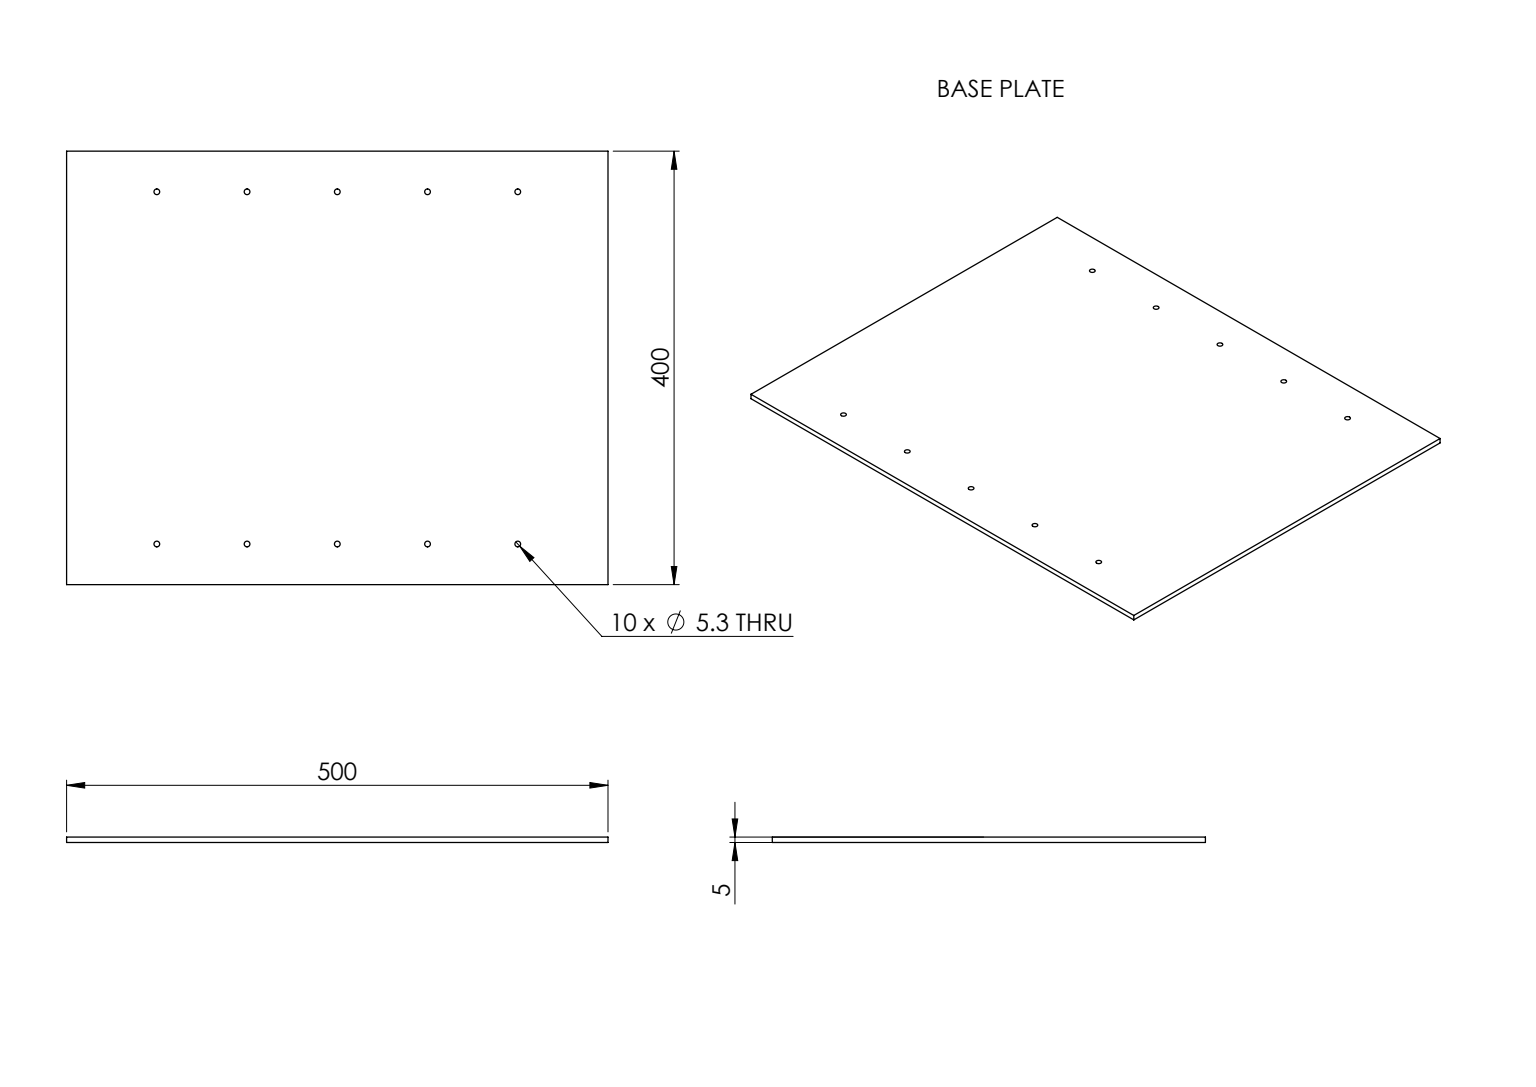
ISO-10303-21;
HEADER;
FILE_DESCRIPTION (('STEP AP214'),
    '1' );
FILE_NAME ('base plate.step',
    '2026-10-24T14:05:44',
    ( '' ),
    ( '' ),
    'SwSTEP 2.0',
    'SolidWorks 2026',
    '' );
FILE_SCHEMA (( 'AUTOMOTIVE_DESIGN' ));
ENDSEC;

DATA;
#1=ORIENTED_EDGE ( 'NONE', *, *, #3686, .F. ) ;
#8=CARTESIAN_POINT ( 'NONE',  ( 53.33333333333330017, -20.00000000000000000, -165.1500000000000625 ) ) ;
#40=ORIENTED_EDGE ( 'NONE', *, *, #976, .T. ) ;
#60=EDGE_LOOP ( 'NONE', ( #5047, #1369, #5230, #2362 ) ) ;
#62=FACE_OUTER_BOUND ( 'NONE', #5362, .T. ) ;
#64=AXIS2_PLACEMENT_3D ( 'NONE', #2945, #3017, #209 ) ;
#88=DIRECTION ( 'NONE',  ( -0.000000000000000000, 1.000000000000000000, -0.000000000000000000 ) ) ;
#107=EDGE_LOOP ( 'NONE', ( #5090, #2760, #2727, #2223 ) ) ;
#119=DIRECTION ( 'NONE',  ( 0.000000000000000000, 0.000000000000000000, 1.000000000000000000 ) ) ;
#126=EDGE_LOOP ( 'NONE', ( #4642, #4899, #6680, #3898 ) ) ;
#139=DIRECTION ( 'NONE',  ( -0.000000000000000000, -1.000000000000000000, -0.000000000000000000 ) ) ;
#143=ADVANCED_FACE ( 'NONE', ( #298 ), #1009, .F. ) ;
#147=EDGE_LOOP ( 'NONE', ( #2986, #2941 ) ) ;
#150=EDGE_CURVE ( 'NONE', #1987, #1784, #6703, .T. ) ;
#153=VERTEX_POINT ( 'NONE', #2555 ) ;
#179=ORIENTED_EDGE ( 'NONE', *, *, #5269, .F. ) ;
#209=DIRECTION ( 'NONE',  ( 0.000000000000000000, 0.000000000000000000, 1.000000000000000000 ) ) ;
#219=ORIENTED_EDGE ( 'NONE', *, *, #5940, .T. ) ;
#235=EDGE_CURVE ( 'NONE', #4841, #4123, #4707, .T. ) ;
#243=DIRECTION ( 'NONE',  ( -0.000000000000000000, -1.000000000000000000, -0.000000000000000000 ) ) ;
#260=EDGE_CURVE ( 'NONE', #6697, #3198, #4705, .T. ) ;
#267=CARTESIAN_POINT ( 'NONE',  ( -30.00000000000002842, -25.00000000000000000, 200.0000000000000000 ) ) ;
#271=VERTEX_POINT ( 'NONE', #4467 ) ;
#277=VECTOR ( 'NONE', #2807, 1000.000000000000000 ) ;
#283=CARTESIAN_POINT ( 'NONE',  ( 219.9999999999999716, -25.00000000000000000, -165.1500000000000625 ) ) ;
#285=CARTESIAN_POINT ( 'NONE',  ( 303.3333333333333144, -25.00000000000000000, -162.5000000000000853 ) ) ;
#287=( NAMED_UNIT ( * ) SI_UNIT ( $, .STERADIAN. ) SOLID_ANGLE_UNIT ( ) );
#298=FACE_OUTER_BOUND ( 'NONE', #2619, .T. ) ;
#302=LINE ( 'NONE', #894, #3741 ) ;
#303=CYLINDRICAL_SURFACE ( 'NONE', #4799, 2.649999999999985700 ) ;
#312=ORIENTED_EDGE ( 'NONE', *, *, #4187, .T. ) ;
#317=CARTESIAN_POINT ( 'NONE',  ( 386.6666666666666288, -20.00000000000000000, 165.1500000000000625 ) ) ;
#333=EDGE_LOOP ( 'NONE', ( #4442, #2385, #6375, #2319 ) ) ;
#334=( GEOMETRIC_REPRESENTATION_CONTEXT ( 3 ) GLOBAL_UNCERTAINTY_ASSIGNED_CONTEXT ( ( #6417 ) ) GLOBAL_UNIT_ASSIGNED_CONTEXT ( ( #4283, #1950, #1436 ) ) REPRESENTATION_CONTEXT ( 'NONE', 'WORKASPACE' ) );
#337=EDGE_CURVE ( 'NONE', #6618, #3696, #5673, .T. ) ;
#338=ORIENTED_EDGE ( 'NONE', *, *, #2679, .T. ) ;
#344=CARTESIAN_POINT ( 'NONE',  ( 136.6666666666666288, -20.00000000000000000, 165.1500000000000625 ) ) ;
#346=CYLINDRICAL_SURFACE ( 'NONE', #6243, 2.649999999999985700 ) ;
#348=EDGE_LOOP ( 'NONE', ( #1624, #5425 ) ) ;
#354=DIRECTION ( 'NONE',  ( 0.000000000000000000, 0.000000000000000000, -1.000000000000000000 ) ) ;
#366=ORIENTED_EDGE ( 'NONE', *, *, #235, .T. ) ;
#381=FACE_OUTER_BOUND ( 'NONE', #2480, .T. ) ;
#391=CARTESIAN_POINT ( 'NONE',  ( -30.00000000000002842, -25.00000000000000000, 200.0000000000000000 ) ) ;
#403=DIRECTION ( 'NONE',  ( -0.000000000000000000, -1.000000000000000000, -0.000000000000000000 ) ) ;
#416=EDGE_CURVE ( 'NONE', #2352, #4993, #2170, .T. ) ;
#420=AXIS2_PLACEMENT_3D ( 'NONE', #1513, #3788, #1169 ) ;
#421=AXIS2_PLACEMENT_3D ( 'NONE', #5145, #5665, #2248 ) ;
#430=EDGE_CURVE ( 'NONE', #5253, #5386, #3873, .T. ) ;
#432=VERTEX_POINT ( 'NONE', #3020 ) ;
#438=CARTESIAN_POINT ( 'NONE',  ( 219.9999999999999716, -20.00000000000000000, -165.1500000000000625 ) ) ;
#440=EDGE_CURVE ( 'NONE', #3349, #7332, #2788, .T. ) ;
#450=VERTEX_POINT ( 'NONE', #1982 ) ;
#459=AXIS2_PLACEMENT_3D ( 'NONE', #4842, #4603, #3459 ) ;
#460=CARTESIAN_POINT ( 'NONE',  ( -30.00000000000002842, -20.00000000000000000, 200.0000000000000000 ) ) ;
#462=EDGE_CURVE ( 'NONE', #1179, #5999, #4944, .T. ) ;
#473=DIRECTION ( 'NONE',  ( 0.000000000000000000, 1.000000000000000000, 0.000000000000000000 ) ) ;
#488=EDGE_LOOP ( 'NONE', ( #3716, #3762 ) ) ;
#513=LINE ( 'NONE', #4964, #4728 ) ;
#517=AXIS2_PLACEMENT_3D ( 'NONE', #2143, #842, #1959 ) ;
#521=EDGE_CURVE ( 'NONE', #1652, #1784, #3123, .T. ) ;
#526=DIRECTION ( 'NONE',  ( -0.000000000000000000, -1.000000000000000000, -0.000000000000000000 ) ) ;
#541=VERTEX_POINT ( 'NONE', #1871 ) ;
#546=AXIS2_PLACEMENT_3D ( 'NONE', #3740, #473, #7159 ) ;
#570=ORIENTED_EDGE ( 'NONE', *, *, #1823, .T. ) ;
#578=ORIENTED_EDGE ( 'NONE', *, *, #7274, .F. ) ;
#579=DIRECTION ( 'NONE',  ( -0.000000000000000000, 1.000000000000000000, -0.000000000000000000 ) ) ;
#582=CARTESIAN_POINT ( 'NONE',  ( 136.6666666666666288, -20.00000000000000000, 162.5000000000000853 ) ) ;
#585=DIRECTION ( 'NONE',  ( 0.000000000000000000, 0.000000000000000000, -1.000000000000000000 ) ) ;
#587=DIRECTION ( 'NONE',  ( -0.000000000000000000, 1.000000000000000000, -0.000000000000000000 ) ) ;
#600=DIRECTION ( 'NONE',  ( -0.000000000000000000, -1.000000000000000000, -0.000000000000000000 ) ) ;
#625=SHAPE_DEFINITION_REPRESENTATION ( #940, #4771 ) ;
#628=DIRECTION ( 'NONE',  ( 0.000000000000000000, 0.000000000000000000, 1.000000000000000000 ) ) ;
#641=ORIENTED_EDGE ( 'NONE', *, *, #1393, .T. ) ;
#647=VERTEX_POINT ( 'NONE', #6436 ) ;
#653=ORIENTED_EDGE ( 'NONE', *, *, #416, .T. ) ;
#658=DIRECTION ( 'NONE',  ( 0.000000000000000000, 0.000000000000000000, -1.000000000000000000 ) ) ;
#659=DIRECTION ( 'NONE',  ( 0.000000000000000000, 1.000000000000000000, 0.000000000000000000 ) ) ;
#672=AXIS2_PLACEMENT_3D ( 'NONE', #2662, #4518, #2775 ) ;
#674=CARTESIAN_POINT ( 'NONE',  ( -30.00000000000002842, -20.00000000000000000, 200.0000000000000000 ) ) ;
#680=EDGE_CURVE ( 'NONE', #5556, #1411, #5423, .T. ) ;
#695=DIRECTION ( 'NONE',  ( 0.000000000000000000, 0.000000000000000000, 1.000000000000000000 ) ) ;
#706=DIRECTION ( 'NONE',  ( 0.000000000000000000, 1.000000000000000000, 0.000000000000000000 ) ) ;
#723=DIRECTION ( 'NONE',  ( -0.000000000000000000, 1.000000000000000000, -0.000000000000000000 ) ) ;
#758=AXIS2_PLACEMENT_3D ( 'NONE', #4531, #139, #4493 ) ;
#763=VERTEX_POINT ( 'NONE', #2931 ) ;
#786=DIRECTION ( 'NONE',  ( -0.000000000000000000, -1.000000000000000000, -0.000000000000000000 ) ) ;
#791=ORIENTED_EDGE ( 'NONE', *, *, #2057, .T. ) ;
#793=CARTESIAN_POINT ( 'NONE',  ( -30.00000000000002842, -20.00000000000000000, 200.0000000000000000 ) ) ;
#795=ORIENTED_EDGE ( 'NONE', *, *, #7297, .F. ) ;
#796=AXIS2_PLACEMENT_3D ( 'NONE', #1331, #817, #2406 ) ;
#799=CARTESIAN_POINT ( 'NONE',  ( 136.6666666666666288, -20.00000000000000000, -162.5000000000000853 ) ) ;
#802=CARTESIAN_POINT ( 'NONE',  ( 53.33333333333330017, -25.00000000000000000, -159.8500000000001080 ) ) ;
#803=DIRECTION ( 'NONE',  ( 0.000000000000000000, 1.000000000000000000, 0.000000000000000000 ) ) ;
#808=CARTESIAN_POINT ( 'NONE',  ( 53.33333333333330017, -20.00000000000000000, -162.5000000000000853 ) ) ;
#817=DIRECTION ( 'NONE',  ( -0.000000000000000000, -1.000000000000000000, -0.000000000000000000 ) ) ;
#822=DIRECTION ( 'NONE',  ( -0.000000000000000000, 1.000000000000000000, -0.000000000000000000 ) ) ;
#835=ORIENTED_EDGE ( 'NONE', *, *, #5690, .T. ) ;
#837=EDGE_LOOP ( 'NONE', ( #3025, #4554, #2784, #5893 ) ) ;
#842=DIRECTION ( 'NONE',  ( 0.000000000000000000, 1.000000000000000000, 0.000000000000000000 ) ) ;
#847=VERTEX_POINT ( 'NONE', #1917 ) ;
#849=EDGE_CURVE ( 'NONE', #1411, #5556, #4851, .T. ) ;
#858=ORIENTED_EDGE ( 'NONE', *, *, #5162, .T. ) ;
#867=DIRECTION ( 'NONE',  ( 0.000000000000000000, 1.000000000000000000, 0.000000000000000000 ) ) ;
#877=SURFACE_STYLE_USAGE ( .BOTH. , #6014 ) ;
#882=CARTESIAN_POINT ( 'NONE',  ( 386.6666666666666288, -25.00000000000000000, -159.8500000000001080 ) ) ;
#891=CIRCLE ( 'NONE', #4830, 2.649999999999985700 ) ;
#894=CARTESIAN_POINT ( 'NONE',  ( 470.0000000000000000, -20.00000000000000000, 200.0000000000000000 ) ) ;
#911=DIRECTION ( 'NONE',  ( -0.000000000000000000, 1.000000000000000000, -0.000000000000000000 ) ) ;
#912=DIRECTION ( 'NONE',  ( 0.000000000000000000, 0.000000000000000000, -1.000000000000000000 ) ) ;
#940=PRODUCT_DEFINITION_SHAPE ( 'NONE', 'NONE',  #1667 ) ;
#950=DIRECTION ( 'NONE',  ( 0.000000000000000000, 0.000000000000000000, -1.000000000000000000 ) ) ;
#976=EDGE_CURVE ( 'NONE', #1043, #7189, #7265, .T. ) ;
#979=AXIS2_PLACEMENT_3D ( 'NONE', #799, #3053, #4229 ) ;
#989=PRODUCT_DEFINITION_CONTEXT ( 'detailed design', #5793, 'design' ) ;
#996=CARTESIAN_POINT ( 'NONE',  ( 219.9999999999999716, -20.00000000000000000, 162.5000000000000853 ) ) ;
#1009=CYLINDRICAL_SURFACE ( 'NONE', #5553, 2.649999999999985700 ) ;
#1010=CARTESIAN_POINT ( 'NONE',  ( 136.6666666666666288, -25.00000000000000000, 162.5000000000000853 ) ) ;
#1015=FACE_BOUND ( 'NONE', #4450, .T. ) ;
#1018=EDGE_CURVE ( 'NONE', #1043, #3333, #7260, .T. ) ;
#1026=EDGE_CURVE ( 'NONE', #271, #6816, #6904, .T. ) ;
#1043=VERTEX_POINT ( 'NONE', #2156 ) ;
#1047=ORIENTED_EDGE ( 'NONE', *, *, #5906, .F. ) ;
#1050=DIRECTION ( 'NONE',  ( 0.000000000000000000, 0.000000000000000000, 1.000000000000000000 ) ) ;
#1054=DIRECTION ( 'NONE',  ( 0.000000000000000000, -0.000000000000000000, 1.000000000000000000 ) ) ;
#1062=ORIENTED_EDGE ( 'NONE', *, *, #6098, .T. ) ;
#1088=AXIS2_PLACEMENT_3D ( 'NONE', #3698, #5427, #3116 ) ;
#1097=LINE ( 'NONE', #3327, #6852 ) ;
#1116=DIRECTION ( 'NONE',  ( 0.000000000000000000, 1.000000000000000000, 0.000000000000000000 ) ) ;
#1119=ORIENTED_EDGE ( 'NONE', *, *, #5813, .F. ) ;
#1121=FACE_BOUND ( 'NONE', #5959, .T. ) ;
#1124=LINE ( 'NONE', #2758, #4238 ) ;
#1131=AXIS2_PLACEMENT_3D ( 'NONE', #6762, #7281, #1465 ) ;
#1134=DIRECTION ( 'NONE',  ( 0.000000000000000000, 1.000000000000000000, 0.000000000000000000 ) ) ;
#1137=CIRCLE ( 'NONE', #6395, 2.649999999999985700 ) ;
#1147=CYLINDRICAL_SURFACE ( 'NONE', #2971, 2.649999999999985700 ) ;
#1148=LINE ( 'NONE', #3417, #4961 ) ;
#1160=AXIS2_PLACEMENT_3D ( 'NONE', #2718, #526, #4490 ) ;
#1163=DIRECTION ( 'NONE',  ( 0.000000000000000000, 1.000000000000000000, 0.000000000000000000 ) ) ;
#1164=EDGE_CURVE ( 'NONE', #5386, #5253, #2926, .T. ) ;
#1169=DIRECTION ( 'NONE',  ( 0.000000000000000000, 0.000000000000000000, -1.000000000000000000 ) ) ;
#1174=DIRECTION ( 'NONE',  ( -0.000000000000000000, 1.000000000000000000, -0.000000000000000000 ) ) ;
#1177=ORIENTED_EDGE ( 'NONE', *, *, #6890, .F. ) ;
#1179=VERTEX_POINT ( 'NONE', #4139 ) ;
#1188=ORIENTED_EDGE ( 'NONE', *, *, #5813, .T. ) ;
#1206=ADVANCED_FACE ( 'NONE', ( #4742 ), #2925, .F. ) ;
#1236=ORIENTED_EDGE ( 'NONE', *, *, #5982, .F. ) ;
#1247=FACE_OUTER_BOUND ( 'NONE', #4443, .T. ) ;
#1258=VECTOR ( 'NONE', #3930, 1000.000000000000000 ) ;
#1261=ORIENTED_EDGE ( 'NONE', *, *, #6825, .F. ) ;
#1269=LINE ( 'NONE', #5767, #1561 ) ;
#1271=LINE ( 'NONE', #3538, #7254 ) ;
#1275=ADVANCED_FACE ( 'NONE', ( #4172 ), #5757, .T. ) ;
#1331=CARTESIAN_POINT ( 'NONE',  ( 386.6666666666666288, -25.00000000000000000, -162.5000000000000853 ) ) ;
#1338=DIRECTION ( 'NONE',  ( 0.000000000000000000, 1.000000000000000000, 0.000000000000000000 ) ) ;
#1340=ORIENTED_EDGE ( 'NONE', *, *, #1164, .T. ) ;
#1347=CARTESIAN_POINT ( 'NONE',  ( 219.9999999999999716, -20.00000000000000000, 165.1500000000000625 ) ) ;
#1349=DIRECTION ( 'NONE',  ( 0.000000000000000000, 0.000000000000000000, 1.000000000000000000 ) ) ;
#1366=UNCERTAINTY_MEASURE_WITH_UNIT (LENGTH_MEASURE( 1.000000000000000082E-05 ), #2021, 'distance_accuracy_value', 'NONE');
#1369=ORIENTED_EDGE ( 'NONE', *, *, #2451, .T. ) ;
#1379=FACE_OUTER_BOUND ( 'NONE', #3006, .T. ) ;
#1393=EDGE_CURVE ( 'NONE', #4485, #3484, #3897, .T. ) ;
#1411=VERTEX_POINT ( 'NONE', #882 ) ;
#1423=EDGE_CURVE ( 'NONE', #3349, #4841, #1557, .T. ) ;
#1424=FACE_OUTER_BOUND ( 'NONE', #3457, .T. ) ;
#1436=( NAMED_UNIT ( * ) SI_UNIT ( $, .STERADIAN. ) SOLID_ANGLE_UNIT ( ) );
#1438=DIRECTION ( 'NONE',  ( 0.000000000000000000, 0.000000000000000000, -1.000000000000000000 ) ) ;
#1446=EDGE_LOOP ( 'NONE', ( #4100, #4125, #4120, #7273 ) ) ;
#1449=CARTESIAN_POINT ( 'NONE',  ( 219.9999999999999716, -20.00000000000000000, 162.5000000000000853 ) ) ;
#1453=EDGE_CURVE ( 'NONE', #2910, #7189, #2090, .T. ) ;
#1456=ORIENTED_EDGE ( 'NONE', *, *, #5758, .T. ) ;
#1465=DIRECTION ( 'NONE',  ( 0.000000000000000000, 0.000000000000000000, -1.000000000000000000 ) ) ;
#1466=EDGE_CURVE ( 'NONE', #647, #3098, #2439, .T. ) ;
#1478=AXIS2_PLACEMENT_3D ( 'NONE', #460, #1163, #1054 ) ;
#1499=VECTOR ( 'NONE', #3835, 1000.000000000000000 ) ;
#1501=FACE_BOUND ( 'NONE', #6434, .T. ) ;
#1504=ORIENTED_EDGE ( 'NONE', *, *, #4187, .F. ) ;
#1508=CARTESIAN_POINT ( 'NONE',  ( 303.3333333333333144, -20.00000000000000000, -159.8500000000001080 ) ) ;
#1510=EDGE_CURVE ( 'NONE', #4492, #3944, #513, .T. ) ;
#1513=CARTESIAN_POINT ( 'NONE',  ( 386.6666666666666288, -25.00000000000000000, -162.5000000000000853 ) ) ;
#1515=EDGE_LOOP ( 'NONE', ( #2970, #4408 ) ) ;
#1533=ORIENTED_EDGE ( 'NONE', *, *, #2575, .F. ) ;
#1540=ORIENTED_EDGE ( 'NONE', *, *, #235, .F. ) ;
#1557=LINE ( 'NONE', #4406, #1499 ) ;
#1561=VECTOR ( 'NONE', #7037, 1000.000000000000000 ) ;
#1569=AXIS2_PLACEMENT_3D ( 'NONE', #7251, #7325, #5370 ) ;
#1577=ORIENTED_EDGE ( 'NONE', *, *, #3686, .T. ) ;
#1578=ORIENTED_EDGE ( 'NONE', *, *, #3283, .T. ) ;
#1585=DIRECTION ( 'NONE',  ( -0.000000000000000000, -1.000000000000000000, -0.000000000000000000 ) ) ;
#1587=VECTOR ( 'NONE', #3164, 1000.000000000000000 ) ;
#1599=CARTESIAN_POINT ( 'NONE',  ( -30.00000000000002842, -25.00000000000000000, -200.0000000000000000 ) ) ;
#1600=ADVANCED_FACE ( 'NONE', ( #5040 ), #5631, .F. ) ;
#1603=AXIS2_PLACEMENT_3D ( 'NONE', #2576, #2138, #7243 ) ;
#1614=ORIENTED_EDGE ( 'NONE', *, *, #2679, .F. ) ;
#1624=ORIENTED_EDGE ( 'NONE', *, *, #337, .T. ) ;
#1643=CIRCLE ( 'NONE', #2578, 2.649999999999985700 ) ;
#1644=DIRECTION ( 'NONE',  ( 0.000000000000000000, 0.000000000000000000, 1.000000000000000000 ) ) ;
#1652=VERTEX_POINT ( 'NONE', #6346 ) ;
#1663=CARTESIAN_POINT ( 'NONE',  ( 53.33333333333330017, -20.00000000000000000, 162.5000000000000853 ) ) ;
#1667=PRODUCT_DEFINITION ( 'UNKNOWN', '', #5185, #989 ) ;
#1687=LINE ( 'NONE', #6264, #5936 ) ;
#1695=DIRECTION ( 'NONE',  ( -0.000000000000000000, 1.000000000000000000, -0.000000000000000000 ) ) ;
#1697=CARTESIAN_POINT ( 'NONE',  ( 219.9999999999999716, -20.00000000000000000, -162.5000000000000853 ) ) ;
#1709=ORIENTED_EDGE ( 'NONE', *, *, #1466, .T. ) ;
#1711=DIRECTION ( 'NONE',  ( 0.000000000000000000, 1.000000000000000000, 0.000000000000000000 ) ) ;
#1729=DIRECTION ( 'NONE',  ( 0.000000000000000000, 1.000000000000000000, 0.000000000000000000 ) ) ;
#1730=EDGE_CURVE ( 'NONE', #5656, #6176, #4084, .T. ) ;
#1740=CARTESIAN_POINT ( 'NONE',  ( -30.00000000000002842, -25.00000000000000000, -200.0000000000000000 ) ) ;
#1746=VECTOR ( 'NONE', #2696, 1000.000000000000000 ) ;
#1748=DIRECTION ( 'NONE',  ( 0.000000000000000000, 0.000000000000000000, 1.000000000000000000 ) ) ;
#1761=ORIENTED_EDGE ( 'NONE', *, *, #6890, .T. ) ;
#1764=DIRECTION ( 'NONE',  ( 0.000000000000000000, 0.000000000000000000, 1.000000000000000000 ) ) ;
#1767=CARTESIAN_POINT ( 'NONE',  ( 136.6666666666666288, -20.00000000000000000, 165.1500000000000625 ) ) ;
#1772=VERTEX_POINT ( 'NONE', #6001 ) ;
#1784=VERTEX_POINT ( 'NONE', #1347 ) ;
#1796=VECTOR ( 'NONE', #7286, 1000.000000000000000 ) ;
#1800=EDGE_CURVE ( 'NONE', #6816, #271, #7127, .T. ) ;
#1803=ORIENTED_EDGE ( 'NONE', *, *, #462, .T. ) ;
#1814=ORIENTED_EDGE ( 'NONE', *, *, #1800, .F. ) ;
#1823=EDGE_CURVE ( 'NONE', #3661, #5128, #4733, .T. ) ;
#1845=AXIS2_PLACEMENT_3D ( 'NONE', #4035, #706, #5800 ) ;
#1860=DIRECTION ( 'NONE',  ( -0.000000000000000000, -1.000000000000000000, -0.000000000000000000 ) ) ;
#1864=EDGE_CURVE ( 'NONE', #7332, #4123, #7277, .T. ) ;
#1871=CARTESIAN_POINT ( 'NONE',  ( 386.6666666666666288, -25.00000000000000000, 159.8500000000001080 ) ) ;
#1895=CARTESIAN_POINT ( 'NONE',  ( 303.3333333333333144, -20.00000000000000000, 159.8500000000001080 ) ) ;
#1898=DIRECTION ( 'NONE',  ( -0.000000000000000000, -1.000000000000000000, -0.000000000000000000 ) ) ;
#1900=CIRCLE ( 'NONE', #6115, 2.649999999999985700 ) ;
#1912=ORIENTED_EDGE ( 'NONE', *, *, #1423, .F. ) ;
#1914=CARTESIAN_POINT ( 'NONE',  ( -30.00000000000002842, -25.00000000000000000, 200.0000000000000000 ) ) ;
#1915=AXIS2_PLACEMENT_3D ( 'NONE', #2600, #4262, #4858 ) ;
#1917=CARTESIAN_POINT ( 'NONE',  ( 53.33333333333330017, -20.00000000000000000, 165.1500000000000625 ) ) ;
#1943=APPLICATION_CONTEXT ( 'automotive_design' ) ;
#1950=( NAMED_UNIT ( * ) PLANE_ANGLE_UNIT ( ) SI_UNIT ( $, .RADIAN. ) );
#1951=FILL_AREA_STYLE ('',( #2546 ) ) ;
#1953=MECHANICAL_DESIGN_GEOMETRIC_PRESENTATION_REPRESENTATION('',(#3392),#4358);
#1959=DIRECTION ( 'NONE',  ( 0.000000000000000000, 0.000000000000000000, -1.000000000000000000 ) ) ;
#1961=ORIENTED_EDGE ( 'NONE', *, *, #5344, .T. ) ;
#1963=AXIS2_PLACEMENT_3D ( 'NONE', #2294, #628, #5829 ) ;
#1970=CYLINDRICAL_SURFACE ( 'NONE', #2320, 2.649999999999985700 ) ;
#1977=PLANE ( 'NONE',  #1088 ) ;
#1980=DIRECTION ( 'NONE',  ( 0.000000000000000000, 1.000000000000000000, 0.000000000000000000 ) ) ;
#1982=CARTESIAN_POINT ( 'NONE',  ( 386.6666666666666288, -25.00000000000000000, 165.1500000000000625 ) ) ;
#1987=VERTEX_POINT ( 'NONE', #4676 ) ;
#1999=ORIENTED_EDGE ( 'NONE', *, *, #6583, .F. ) ;
#2010=CARTESIAN_POINT ( 'NONE',  ( 303.3333333333333144, -20.00000000000000000, -162.5000000000000853 ) ) ;
#2012=FACE_OUTER_BOUND ( 'NONE', #6212, .T. ) ;
#2021=( LENGTH_UNIT ( ) NAMED_UNIT ( * ) SI_UNIT ( .MILLI., .METRE. ) );
#2029=PLANE ( 'NONE',  #6297 ) ;
#2037=DIRECTION ( 'NONE',  ( 0.000000000000000000, 0.000000000000000000, -1.000000000000000000 ) ) ;
#2040=CARTESIAN_POINT ( 'NONE',  ( 53.33333333333330017, -20.00000000000000000, 162.5000000000000853 ) ) ;
#2046=EDGE_CURVE ( 'NONE', #647, #7294, #1271, .T. ) ;
#2057=EDGE_CURVE ( 'NONE', #5128, #6618, #1687, .T. ) ;
#2060=CARTESIAN_POINT ( 'NONE',  ( -30.00000000000002842, -20.00000000000000000, 200.0000000000000000 ) ) ;
#2075=CIRCLE ( 'NONE', #6508, 2.649999999999985700 ) ;
#2090=CIRCLE ( 'NONE', #672, 2.649999999999985700 ) ;
#2092=FACE_BOUND ( 'NONE', #2505, .T. ) ;
#2104=EDGE_CURVE ( 'NONE', #2352, #2399, #3287, .T. ) ;
#2113=DIRECTION ( 'NONE',  ( -0.000000000000000000, 1.000000000000000000, -0.000000000000000000 ) ) ;
#2123=LINE ( 'NONE', #8, #6736 ) ;
#2132=EDGE_LOOP ( 'NONE', ( #578, #5329, #6288, #6562 ) ) ;
#2135=CARTESIAN_POINT ( 'NONE',  ( 219.9999999999999716, -25.00000000000000000, 162.5000000000000853 ) ) ;
#2137=DIRECTION ( 'NONE',  ( -0.000000000000000000, -0.000000000000000000, -1.000000000000000000 ) ) ;
#2138=DIRECTION ( 'NONE',  ( -0.000000000000000000, 1.000000000000000000, -0.000000000000000000 ) ) ;
#2139=ORIENTED_EDGE ( 'NONE', *, *, #5690, .F. ) ;
#2143=CARTESIAN_POINT ( 'NONE',  ( 219.9999999999999716, -20.00000000000000000, -162.5000000000000853 ) ) ;
#2145=( LENGTH_UNIT ( ) NAMED_UNIT ( * ) SI_UNIT ( .MILLI., .METRE. ) );
#2146=CYLINDRICAL_SURFACE ( 'NONE', #5290, 2.649999999999985700 ) ;
#2147=ORIENTED_EDGE ( 'NONE', *, *, #5344, .F. ) ;
#2149=EDGE_CURVE ( 'NONE', #3484, #4485, #5187, .T. ) ;
#2153=CARTESIAN_POINT ( 'NONE',  ( 303.3333333333333144, -25.00000000000000000, 165.1500000000000625 ) ) ;
#2156=CARTESIAN_POINT ( 'NONE',  ( 136.6666666666666288, -25.00000000000000000, 159.8500000000001080 ) ) ;
#2159=PLANE ( 'NONE',  #1478 ) ;
#2170=LINE ( 'NONE', #438, #6628 ) ;
#2189=AXIS2_PLACEMENT_3D ( 'NONE', #6987, #4093, #2950 ) ;
#2195=CARTESIAN_POINT ( 'NONE',  ( 386.6666666666666288, -20.00000000000000000, 162.5000000000000853 ) ) ;
#2196=CARTESIAN_POINT ( 'NONE',  ( 386.6666666666666288, -25.00000000000000000, -165.1500000000000625 ) ) ;
#2201=AXIS2_PLACEMENT_3D ( 'NONE', #2040, #822, #6674 ) ;
#2215=ORIENTED_EDGE ( 'NONE', *, *, #2149, .F. ) ;
#2216=AXIS2_PLACEMENT_3D ( 'NONE', #6208, #6238, #5117 ) ;
#2223=ORIENTED_EDGE ( 'NONE', *, *, #5444, .T. ) ;
#2224=ORIENTED_EDGE ( 'NONE', *, *, #4880, .F. ) ;
#2242=ADVANCED_FACE ( 'NONE', ( #3596 ), #4135, .F. ) ;
#2248=DIRECTION ( 'NONE',  ( 0.000000000000000000, 0.000000000000000000, 1.000000000000000000 ) ) ;
#2251=CARTESIAN_POINT ( 'NONE',  ( 386.6666666666666288, -20.00000000000000000, -162.5000000000000853 ) ) ;
#2268=EDGE_CURVE ( 'NONE', #7332, #3349, #4477, .T. ) ;
#2283=CARTESIAN_POINT ( 'NONE',  ( 219.9999999999999716, -20.00000000000000000, 162.5000000000000853 ) ) ;
#2294=CARTESIAN_POINT ( 'NONE',  ( 0.000000000000000000, 0.000000000000000000, 0.000000000000000000 ) ) ;
#2295=DIRECTION ( 'NONE',  ( -0.000000000000000000, -1.000000000000000000, -0.000000000000000000 ) ) ;
#2306=CIRCLE ( 'NONE', #5552, 2.649999999999985700 ) ;
#2318=DIRECTION ( 'NONE',  ( -0.000000000000000000, -1.000000000000000000, -0.000000000000000000 ) ) ;
#2319=ORIENTED_EDGE ( 'NONE', *, *, #3511, .T. ) ;
#2320=AXIS2_PLACEMENT_3D ( 'NONE', #1449, #6586, #7269 ) ;
#2337=ORIENTED_EDGE ( 'NONE', *, *, #440, .T. ) ;
#2342=EDGE_LOOP ( 'NONE', ( #5280, #338, #5791, #2215 ) ) ;
#2345=CARTESIAN_POINT ( 'NONE',  ( 219.9999999999999716, -25.00000000000000000, -162.5000000000000853 ) ) ;
#2352=VERTEX_POINT ( 'NONE', #283 ) ;
#2362=ORIENTED_EDGE ( 'NONE', *, *, #3744, .F. ) ;
#2369=LINE ( 'NONE', #674, #7245 ) ;
#2372=ORIENTED_EDGE ( 'NONE', *, *, #2268, .T. ) ;
#2385=ORIENTED_EDGE ( 'NONE', *, *, #5609, .F. ) ;
#2399=VERTEX_POINT ( 'NONE', #3637 ) ;
#2406=DIRECTION ( 'NONE',  ( 0.000000000000000000, 0.000000000000000000, -1.000000000000000000 ) ) ;
#2415=CARTESIAN_POINT ( 'NONE',  ( 219.9999999999999716, -20.00000000000000000, -162.5000000000000853 ) ) ;
#2422=CIRCLE ( 'NONE', #3244, 2.649999999999985700 ) ;
#2439=CIRCLE ( 'NONE', #2216, 2.649999999999985700 ) ;
#2442=ORIENTED_EDGE ( 'NONE', *, *, #1018, .F. ) ;
#2451=EDGE_CURVE ( 'NONE', #541, #4054, #6124, .T. ) ;
#2454=CARTESIAN_POINT ( 'NONE',  ( 470.0000000000000000, -25.00000000000000000, -200.0000000000000000 ) ) ;
#2465=CARTESIAN_POINT ( 'NONE',  ( 219.9999999999999716, -25.00000000000000000, -162.5000000000000853 ) ) ;
#2473=EDGE_CURVE ( 'NONE', #5556, #5386, #5468, .T. ) ;
#2474=DIRECTION ( 'NONE',  ( 0.000000000000000000, 0.000000000000000000, -1.000000000000000000 ) ) ;
#2479=DIRECTION ( 'NONE',  ( -0.000000000000000000, 1.000000000000000000, -0.000000000000000000 ) ) ;
#2480=EDGE_LOOP ( 'NONE', ( #5419, #6968, #5576, #2908 ) ) ;
#2483=ADVANCED_FACE ( 'NONE', ( #7161 ), #6648, .F. ) ;
#2499=CARTESIAN_POINT ( 'NONE',  ( 53.33333333333330017, -25.00000000000000000, -162.5000000000000853 ) ) ;
#2505=EDGE_LOOP ( 'NONE', ( #6305, #6043 ) ) ;
#2519=CIRCLE ( 'NONE', #2881, 2.649999999999985700 ) ;
#2521=CARTESIAN_POINT ( 'NONE',  ( 303.3333333333333144, -25.00000000000000000, -162.5000000000000853 ) ) ;
#2531=DIRECTION ( 'NONE',  ( -0.000000000000000000, -1.000000000000000000, -0.000000000000000000 ) ) ;
#2538=EDGE_LOOP ( 'NONE', ( #6113, #2147 ) ) ;
#2546=FILL_AREA_STYLE_COLOUR ( '', #5195 ) ;
#2550=VECTOR ( 'NONE', #4413, 1000.000000000000000 ) ;
#2555=CARTESIAN_POINT ( 'NONE',  ( 219.9999999999999716, -20.00000000000000000, -159.8500000000001080 ) ) ;
#2575=EDGE_CURVE ( 'NONE', #5128, #3661, #3001, .T. ) ;
#2576=CARTESIAN_POINT ( 'NONE',  ( 136.6666666666666288, -20.00000000000000000, 162.5000000000000853 ) ) ;
#2578=AXIS2_PLACEMENT_3D ( 'NONE', #285, #600, #6997 ) ;
#2580=LINE ( 'NONE', #2060, #1796 ) ;
#2585=CARTESIAN_POINT ( 'NONE',  ( 53.33333333333330017, -25.00000000000000000, 165.1500000000000625 ) ) ;
#2600=CARTESIAN_POINT ( 'NONE',  ( 386.6666666666666288, -20.00000000000000000, -162.5000000000000853 ) ) ;
#2605=FACE_BOUND ( 'NONE', #6924, .T. ) ;
#2612=ADVANCED_FACE ( 'NONE', ( #4579 ), #5741, .F. ) ;
#2614=CARTESIAN_POINT ( 'NONE',  ( 386.6666666666666288, -20.00000000000000000, -165.1500000000000625 ) ) ;
#2615=DIRECTION ( 'NONE',  ( -0.000000000000000000, 1.000000000000000000, -0.000000000000000000 ) ) ;
#2619=EDGE_LOOP ( 'NONE', ( #6575, #4826, #7096, #4865 ) ) ;
#2620=CARTESIAN_POINT ( 'NONE',  ( -30.00000000000002842, -25.00000000000000000, 200.0000000000000000 ) ) ;
#2646=EDGE_LOOP ( 'NONE', ( #4134, #1236, #5721, #858 ) ) ;
#2650=ADVANCED_FACE ( 'NONE', ( #3474 ), #5627, .F. ) ;
#2655=CARTESIAN_POINT ( 'NONE',  ( 136.6666666666666288, -20.00000000000000000, -162.5000000000000853 ) ) ;
#2662=CARTESIAN_POINT ( 'NONE',  ( 136.6666666666666288, -20.00000000000000000, 162.5000000000000853 ) ) ;
#2679=EDGE_CURVE ( 'NONE', #5999, #1179, #2306, .T. ) ;
#2681=VECTOR ( 'NONE', #1338, 1000.000000000000000 ) ;
#2690=FACE_BOUND ( 'NONE', #4445, .T. ) ;
#2696=DIRECTION ( 'NONE',  ( -0.000000000000000000, 1.000000000000000000, -0.000000000000000000 ) ) ;
#2706=FACE_OUTER_BOUND ( 'NONE', #5833, .T. ) ;
#2708=PRESENTATION_STYLE_ASSIGNMENT (( #877 ) ) ;
#2710=ADVANCED_BREP_SHAPE_REPRESENTATION ( '', ( #5676, #1963 ), #6040 ) ;
#2712=ORIENTED_EDGE ( 'NONE', *, *, #440, .F. ) ;
#2718=CARTESIAN_POINT ( 'NONE',  ( 386.6666666666666288, -20.00000000000000000, -162.5000000000000853 ) ) ;
#2727=ORIENTED_EDGE ( 'NONE', *, *, #7004, .T. ) ;
#2752=CIRCLE ( 'NONE', #1569, 2.649999999999985700 ) ;
#2758=CARTESIAN_POINT ( 'NONE',  ( 136.6666666666666288, -20.00000000000000000, -159.8500000000001080 ) ) ;
#2760=ORIENTED_EDGE ( 'NONE', *, *, #4565, .F. ) ;
#2775=DIRECTION ( 'NONE',  ( 0.000000000000000000, 0.000000000000000000, 1.000000000000000000 ) ) ;
#2784=ORIENTED_EDGE ( 'NONE', *, *, #337, .F. ) ;
#2788=CIRCLE ( 'NONE', #5304, 2.649999999999985700 ) ;
#2807=DIRECTION ( 'NONE',  ( 0.000000000000000000, 1.000000000000000000, 0.000000000000000000 ) ) ;
#2812=ORIENTED_EDGE ( 'NONE', *, *, #260, .F. ) ;
#2816=FACE_OUTER_BOUND ( 'NONE', #1446, .T. ) ;
#2823=LINE ( 'NONE', #1599, #2550 ) ;
#2824=EDGE_CURVE ( 'NONE', #4123, #4841, #2422, .T. ) ;
#2838=DIRECTION ( 'NONE',  ( 0.000000000000000000, 0.000000000000000000, 1.000000000000000000 ) ) ;
#2841=EDGE_LOOP ( 'NONE', ( #7003, #5682 ) ) ;
#2847=DIRECTION ( 'NONE',  ( 0.000000000000000000, 1.000000000000000000, 0.000000000000000000 ) ) ;
#2851=LINE ( 'NONE', #6248, #5439 ) ;
#2857=AXIS2_PLACEMENT_3D ( 'NONE', #6864, #5108, #3437 ) ;
#2868=DIRECTION ( 'NONE',  ( -0.000000000000000000, 1.000000000000000000, -0.000000000000000000 ) ) ;
#2874=VERTEX_POINT ( 'NONE', #793 ) ;
#2881=AXIS2_PLACEMENT_3D ( 'NONE', #2135, #4308, #6597 ) ;
#2891=AXIS2_PLACEMENT_3D ( 'NONE', #7219, #4375, #1050 ) ;
#2908=ORIENTED_EDGE ( 'NONE', *, *, #260, .T. ) ;
#2910=VERTEX_POINT ( 'NONE', #344 ) ;
#2925=PLANE ( 'NONE',  #7133 ) ;
#2926=CIRCLE ( 'NONE', #1160, 2.649999999999985700 ) ;
#2927=EDGE_LOOP ( 'NONE', ( #1912, #5411, #4848, #6287 ) ) ;
#2929=DIRECTION ( 'NONE',  ( 1.000000000000000000, 0.000000000000000000, 0.000000000000000000 ) ) ;
#2931=CARTESIAN_POINT ( 'NONE',  ( 219.9999999999999716, -25.00000000000000000, 159.8500000000001080 ) ) ;
#2941=ORIENTED_EDGE ( 'NONE', *, *, #1018, .T. ) ;
#2945=CARTESIAN_POINT ( 'NONE',  ( 303.3333333333333144, -20.00000000000000000, 162.5000000000000853 ) ) ;
#2949=ADVANCED_FACE ( 'NONE', ( #5383, #6712, #2690, #2092, #7152, #2605, #4386, #3197, #4900, #1501, #381 ), #4338, .F. ) ;
#2950=DIRECTION ( 'NONE',  ( 0.000000000000000000, 0.000000000000000000, 1.000000000000000000 ) ) ;
#2970=ORIENTED_EDGE ( 'NONE', *, *, #5162, .F. ) ;
#2971=AXIS2_PLACEMENT_3D ( 'NONE', #1697, #3985, #658 ) ;
#2977=DIRECTION ( 'NONE',  ( 0.000000000000000000, 0.000000000000000000, 1.000000000000000000 ) ) ;
#2986=ORIENTED_EDGE ( 'NONE', *, *, #6992, .T. ) ;
#2998=AXIS2_PLACEMENT_3D ( 'NONE', #7053, #803, #695 ) ;
#3001=CIRCLE ( 'NONE', #3993, 2.649999999999985700 ) ;
#3006=EDGE_LOOP ( 'NONE', ( #5374, #6418, #1814, #5447 ) ) ;
#3016=CARTESIAN_POINT ( 'NONE',  ( 53.33333333333330017, -20.00000000000000000, -159.8500000000001080 ) ) ;
#3017=DIRECTION ( 'NONE',  ( -0.000000000000000000, 1.000000000000000000, -0.000000000000000000 ) ) ;
#3020=CARTESIAN_POINT ( 'NONE',  ( 303.3333333333333144, -25.00000000000000000, -159.8500000000001080 ) ) ;
#3025=ORIENTED_EDGE ( 'NONE', *, *, #2575, .T. ) ;
#3031=DIRECTION ( 'NONE',  ( -1.000000000000000000, 0.000000000000000000, -0.000000000000000000 ) ) ;
#3052=ADVANCED_FACE ( 'NONE', ( #3759 ), #2146, .F. ) ;
#3053=DIRECTION ( 'NONE',  ( -0.000000000000000000, -1.000000000000000000, -0.000000000000000000 ) ) ;
#3065=( NAMED_UNIT ( * ) PLANE_ANGLE_UNIT ( ) SI_UNIT ( $, .RADIAN. ) );
#3076=DIRECTION ( 'NONE',  ( 0.000000000000000000, 1.000000000000000000, 0.000000000000000000 ) ) ;
#3098=VERTEX_POINT ( 'NONE', #2585 ) ;
#3102=DIRECTION ( 'NONE',  ( -0.000000000000000000, 1.000000000000000000, -0.000000000000000000 ) ) ;
#3107=CYLINDRICAL_SURFACE ( 'NONE', #1915, 2.649999999999985700 ) ;
#3116=DIRECTION ( 'NONE',  ( -0.000000000000000000, 0.000000000000000000, -1.000000000000000000 ) ) ;
#3121=VECTOR ( 'NONE', #3076, 1000.000000000000000 ) ;
#3122=AXIS2_PLACEMENT_3D ( 'NONE', #3310, #1116, #7262 ) ;
#3123=CIRCLE ( 'NONE', #6872, 2.649999999999985700 ) ;
#3128=DIRECTION ( 'NONE',  ( 0.000000000000000000, 0.000000000000000000, 1.000000000000000000 ) ) ;
#3134=ORIENTED_EDGE ( 'NONE', *, *, #6128, .F. ) ;
#3145=VECTOR ( 'NONE', #2479, 1000.000000000000000 ) ;
#3161=EDGE_LOOP ( 'NONE', ( #6505, #1614 ) ) ;
#3164=DIRECTION ( 'NONE',  ( 0.000000000000000000, 1.000000000000000000, 0.000000000000000000 ) ) ;
#3165=LINE ( 'NONE', #7279, #3500 ) ;
#3193=CARTESIAN_POINT ( 'NONE',  ( -30.00000000000002842, -25.00000000000000000, 200.0000000000000000 ) ) ;
#3197=FACE_BOUND ( 'NONE', #4007, .T. ) ;
#3198=VERTEX_POINT ( 'NONE', #1740 ) ;
#3204=DIRECTION ( 'NONE',  ( 0.000000000000000000, 1.000000000000000000, 0.000000000000000000 ) ) ;
#3210=DIRECTION ( 'NONE',  ( -0.000000000000000000, 1.000000000000000000, -0.000000000000000000 ) ) ;
#3240=DIRECTION ( 'NONE',  ( 0.000000000000000000, 0.000000000000000000, -1.000000000000000000 ) ) ;
#3244=AXIS2_PLACEMENT_3D ( 'NONE', #4185, #5846, #5960 ) ;
#3251=DIRECTION ( 'NONE',  ( 0.000000000000000000, 1.000000000000000000, 0.000000000000000000 ) ) ;
#3259=AXIS2_PLACEMENT_3D ( 'NONE', #4309, #4395, #6161 ) ;
#3267=CARTESIAN_POINT ( 'NONE',  ( 219.9999999999999716, -20.00000000000000000, 165.1500000000000625 ) ) ;
#3274=FACE_OUTER_BOUND ( 'NONE', #107, .T. ) ;
#3279=VECTOR ( 'NONE', #5818, 1000.000000000000000 ) ;
#3280=VERTEX_POINT ( 'NONE', #4796 ) ;
#3283=EDGE_CURVE ( 'NONE', #541, #450, #5901, .T. ) ;
#3287=CIRCLE ( 'NONE', #4250, 2.649999999999985700 ) ;
#3310=CARTESIAN_POINT ( 'NONE',  ( 136.6666666666666288, -20.00000000000000000, -162.5000000000000853 ) ) ;
#3327=CARTESIAN_POINT ( 'NONE',  ( 386.6666666666666288, -20.00000000000000000, 165.1500000000000625 ) ) ;
#3331=DIRECTION ( 'NONE',  ( 0.000000000000000000, 0.000000000000000000, -1.000000000000000000 ) ) ;
#3333=VERTEX_POINT ( 'NONE', #4690 ) ;
#3334=DIRECTION ( 'NONE',  ( 0.000000000000000000, 0.000000000000000000, 1.000000000000000000 ) ) ;
#3335=DIRECTION ( 'NONE',  ( -0.000000000000000000, -0.000000000000000000, -1.000000000000000000 ) ) ;
#3346=FACE_OUTER_BOUND ( 'NONE', #837, .T. ) ;
#3349=VERTEX_POINT ( 'NONE', #3554 ) ;
#3353=CARTESIAN_POINT ( 'NONE',  ( 303.3333333333333144, -20.00000000000000000, -165.1500000000000625 ) ) ;
#3361=CARTESIAN_POINT ( 'NONE',  ( 303.3333333333333144, -20.00000000000000000, 165.1500000000000625 ) ) ;
#3375=AXIS2_PLACEMENT_3D ( 'NONE', #267, #7116, #6677 ) ;
#3392=STYLED_ITEM ( 'NONE', ( #2708 ), #2710 ) ;
#3394=FACE_BOUND ( 'NONE', #3889, .T. ) ;
#3417=CARTESIAN_POINT ( 'NONE',  ( 53.33333333333330017, -20.00000000000000000, -159.8500000000001080 ) ) ;
#3437=DIRECTION ( 'NONE',  ( 0.000000000000000000, 0.000000000000000000, 1.000000000000000000 ) ) ;
#3457=EDGE_LOOP ( 'NONE', ( #795, #4640, #1761, #5189 ) ) ;
#3459=DIRECTION ( 'NONE',  ( 0.000000000000000000, 0.000000000000000000, 1.000000000000000000 ) ) ;
#3474=FACE_OUTER_BOUND ( 'NONE', #2927, .T. ) ;
#3479=DIRECTION ( 'NONE',  ( -0.000000000000000000, 1.000000000000000000, -0.000000000000000000 ) ) ;
#3481=CIRCLE ( 'NONE', #4454, 2.649999999999985700 ) ;
#3484=VERTEX_POINT ( 'NONE', #3016 ) ;
#3500=VECTOR ( 'NONE', #1980, 1000.000000000000000 ) ;
#3511=EDGE_CURVE ( 'NONE', #847, #7294, #3598, .T. ) ;
#3522=AXIS2_PLACEMENT_3D ( 'NONE', #808, #403, #1438 ) ;
#3534=CIRCLE ( 'NONE', #459, 2.649999999999985700 ) ;
#3538=CARTESIAN_POINT ( 'NONE',  ( 53.33333333333330017, -20.00000000000000000, 159.8500000000001080 ) ) ;
#3544=PRODUCT ( 'base plate', 'base plate', '', ( #3959 ) ) ;
#3552=CARTESIAN_POINT ( 'NONE',  ( 219.9999999999999716, -20.00000000000000000, -159.8500000000001080 ) ) ;
#3554=CARTESIAN_POINT ( 'NONE',  ( 303.3333333333333144, -25.00000000000000000, 159.8500000000001080 ) ) ;
#3562=EDGE_CURVE ( 'NONE', #432, #271, #5464, .T. ) ;
#3596=FACE_OUTER_BOUND ( 'NONE', #60, .T. ) ;
#3598=CIRCLE ( 'NONE', #6740, 2.649999999999985700 ) ;
#3599=CARTESIAN_POINT ( 'NONE',  ( 0.000000000000000000, 0.000000000000000000, -200.0000000000000000 ) ) ;
#3603=ORIENTED_EDGE ( 'NONE', *, *, #1864, .F. ) ;
#3610=ORIENTED_EDGE ( 'NONE', *, *, #7060, .T. ) ;
#3621=EDGE_LOOP ( 'NONE', ( #1533, #4079 ) ) ;
#3623=AXIS2_PLACEMENT_3D ( 'NONE', #6343, #1729, #3331 ) ;
#3628=CIRCLE ( 'NONE', #3259, 2.649999999999985700 ) ;
#3633=DIRECTION ( 'NONE',  ( 0.000000000000000000, 1.000000000000000000, 0.000000000000000000 ) ) ;
#3637=CARTESIAN_POINT ( 'NONE',  ( 219.9999999999999716, -25.00000000000000000, -159.8500000000001080 ) ) ;
#3661=VERTEX_POINT ( 'NONE', #4394 ) ;
#3686=EDGE_CURVE ( 'NONE', #1987, #763, #2519, .T. ) ;
#3696=VERTEX_POINT ( 'NONE', #5737 ) ;
#3698=CARTESIAN_POINT ( 'NONE',  ( 470.0000000000000000, -20.00000000000000000, 200.0000000000000000 ) ) ;
#3712=EDGE_CURVE ( 'NONE', #1411, #5253, #4614, .T. ) ;
#3716=ORIENTED_EDGE ( 'NONE', *, *, #1800, .T. ) ;
#3720=DIRECTION ( 'NONE',  ( 0.000000000000000000, 1.000000000000000000, 0.000000000000000000 ) ) ;
#3728=ORIENTED_EDGE ( 'NONE', *, *, #5596, .F. ) ;
#3740=CARTESIAN_POINT ( 'NONE',  ( 136.6666666666666288, -20.00000000000000000, -162.5000000000000853 ) ) ;
#3741=VECTOR ( 'NONE', #6584, 1000.000000000000000 ) ;
#3744=EDGE_CURVE ( 'NONE', #450, #6179, #1097, .T. ) ;
#3759=FACE_OUTER_BOUND ( 'NONE', #2646, .T. ) ;
#3762=ORIENTED_EDGE ( 'NONE', *, *, #1026, .T. ) ;
#3771=CYLINDRICAL_SURFACE ( 'NONE', #6029, 2.649999999999985700 ) ;
#3776=ORIENTED_EDGE ( 'NONE', *, *, #1393, .F. ) ;
#3780=AXIS2_PLACEMENT_3D ( 'NONE', #6782, #2295, #6296 ) ;
#3788=DIRECTION ( 'NONE',  ( -0.000000000000000000, -1.000000000000000000, -0.000000000000000000 ) ) ;
#3793=ADVANCED_FACE ( 'NONE', ( #5707 ), #4043, .F. ) ;
#3797=ORIENTED_EDGE ( 'NONE', *, *, #2104, .F. ) ;
#3804=DIRECTION ( 'NONE',  ( -1.000000000000000000, 0.000000000000000000, 0.000000000000000000 ) ) ;
#3835=DIRECTION ( 'NONE',  ( -0.000000000000000000, 1.000000000000000000, -0.000000000000000000 ) ) ;
#3838=EDGE_LOOP ( 'NONE', ( #7210, #1, #5824, #1188 ) ) ;
#3844=DIRECTION ( 'NONE',  ( 0.000000000000000000, 0.000000000000000000, -1.000000000000000000 ) ) ;
#3850=FACE_OUTER_BOUND ( 'NONE', #4371, .T. ) ;
#3851=CYLINDRICAL_SURFACE ( 'NONE', #2201, 2.649999999999985700 ) ;
#3866=DIRECTION ( 'NONE',  ( -0.000000000000000000, -1.000000000000000000, -0.000000000000000000 ) ) ;
#3873=CIRCLE ( 'NONE', #1131, 2.649999999999985700 ) ;
#3889=EDGE_LOOP ( 'NONE', ( #1119, #4269 ) ) ;
#3890=EDGE_CURVE ( 'NONE', #432, #1772, #5166, .T. ) ;
#3897=CIRCLE ( 'NONE', #3522, 2.649999999999985700 ) ;
#3898=ORIENTED_EDGE ( 'NONE', *, *, #1453, .T. ) ;
#3928=CARTESIAN_POINT ( 'NONE',  ( 53.33333333333330017, -25.00000000000000000, 162.5000000000000853 ) ) ;
#3930=DIRECTION ( 'NONE',  ( 0.000000000000000000, -1.000000000000000000, 0.000000000000000000 ) ) ;
#3944=VERTEX_POINT ( 'NONE', #2454 ) ;
#3957=ORIENTED_EDGE ( 'NONE', *, *, #1423, .T. ) ;
#3959=PRODUCT_CONTEXT ( 'NONE', #1943, 'mechanical' ) ;
#3962=ADVANCED_FACE ( 'NONE', ( #5956 ), #303, .F. ) ;
#3967=AXIS2_PLACEMENT_3D ( 'NONE', #2283, #587, #1764 ) ;
#3985=DIRECTION ( 'NONE',  ( 0.000000000000000000, 1.000000000000000000, 0.000000000000000000 ) ) ;
#3992=VECTOR ( 'NONE', #2137, 1000.000000000000000 ) ;
#3993=AXIS2_PLACEMENT_3D ( 'NONE', #5507, #1585, #950 ) ;
#4001=ORIENTED_EDGE ( 'NONE', *, *, #2046, .T. ) ;
#4007=EDGE_LOOP ( 'NONE', ( #1577, #312 ) ) ;
#4010=AXIS2_PLACEMENT_3D ( 'NONE', #2195, #6785, #1644 ) ;
#4035=CARTESIAN_POINT ( 'NONE',  ( 136.6666666666666288, -25.00000000000000000, 162.5000000000000853 ) ) ;
#4043=CYLINDRICAL_SURFACE ( 'NONE', #4200, 2.649999999999985700 ) ;
#4054=VERTEX_POINT ( 'NONE', #7148 ) ;
#4065=ADVANCED_FACE ( 'NONE', ( #3850 ), #3107, .F. ) ;
#4069=CIRCLE ( 'NONE', #5382, 2.649999999999985700 ) ;
#4079=ORIENTED_EDGE ( 'NONE', *, *, #1823, .F. ) ;
#4084=LINE ( 'NONE', #6380, #3279 ) ;
#4093=DIRECTION ( 'NONE',  ( 0.000000000000000000, 1.000000000000000000, 0.000000000000000000 ) ) ;
#4100=ORIENTED_EDGE ( 'NONE', *, *, #2104, .T. ) ;
#4120=ORIENTED_EDGE ( 'NONE', *, *, #6581, .F. ) ;
#4123=VERTEX_POINT ( 'NONE', #4849 ) ;
#4125=ORIENTED_EDGE ( 'NONE', *, *, #5906, .T. ) ;
#4134=ORIENTED_EDGE ( 'NONE', *, *, #2451, .F. ) ;
#4135=CYLINDRICAL_SURFACE ( 'NONE', #4010, 2.649999999999985700 ) ;
#4139=CARTESIAN_POINT ( 'NONE',  ( 53.33333333333330017, -25.00000000000000000, -165.1500000000000625 ) ) ;
#4142=ADVANCED_FACE ( 'NONE', ( #2706 ), #4776, .F. ) ;
#4172=FACE_OUTER_BOUND ( 'NONE', #2132, .T. ) ;
#4185=CARTESIAN_POINT ( 'NONE',  ( 303.3333333333333144, -20.00000000000000000, 162.5000000000000853 ) ) ;
#4187=EDGE_CURVE ( 'NONE', #763, #1987, #2752, .T. ) ;
#4194=DIRECTION ( 'NONE',  ( 0.000000000000000000, 0.000000000000000000, -1.000000000000000000 ) ) ;
#4195=CIRCLE ( 'NONE', #979, 2.649999999999985700 ) ;
#4200=AXIS2_PLACEMENT_3D ( 'NONE', #582, #2868, #2838 ) ;
#4207=UNCERTAINTY_MEASURE_WITH_UNIT (LENGTH_MEASURE( 1.000000000000000082E-05 ), #2145, 'distance_accuracy_value', 'NONE');
#4218=AXIS2_PLACEMENT_3D ( 'NONE', #2655, #3866, #354 ) ;
#4227=ORIENTED_EDGE ( 'NONE', *, *, #3712, .T. ) ;
#4229=DIRECTION ( 'NONE',  ( 0.000000000000000000, 0.000000000000000000, -1.000000000000000000 ) ) ;
#4238=VECTOR ( 'NONE', #6189, 1000.000000000000000 ) ;
#4250=AXIS2_PLACEMENT_3D ( 'NONE', #2345, #7007, #4716 ) ;
#4256=AXIS2_PLACEMENT_3D ( 'NONE', #1010, #6892, #1748 ) ;
#4259=ORIENTED_EDGE ( 'NONE', *, *, #2149, .T. ) ;
#4262=DIRECTION ( 'NONE',  ( 0.000000000000000000, 1.000000000000000000, 0.000000000000000000 ) ) ;
#4269=ORIENTED_EDGE ( 'NONE', *, *, #521, .F. ) ;
#4276=DIRECTION ( 'NONE',  ( 0.000000000000000000, 0.000000000000000000, 1.000000000000000000 ) ) ;
#4283=( LENGTH_UNIT ( ) NAMED_UNIT ( * ) SI_UNIT ( .MILLI., .METRE. ) );
#4284=SURFACE_STYLE_FILL_AREA ( #1951 ) ;
#4289=CARTESIAN_POINT ( 'NONE',  ( 136.6666666666666288, -20.00000000000000000, 159.8500000000001080 ) ) ;
#4301=CIRCLE ( 'NONE', #2857, 2.649999999999985700 ) ;
#4308=DIRECTION ( 'NONE',  ( 0.000000000000000000, 1.000000000000000000, 0.000000000000000000 ) ) ;
#4309=CARTESIAN_POINT ( 'NONE',  ( 219.9999999999999716, -20.00000000000000000, -162.5000000000000853 ) ) ;
#4338=PLANE ( 'NONE',  #3375 ) ;
#4358=( GEOMETRIC_REPRESENTATION_CONTEXT ( 3 ) GLOBAL_UNCERTAINTY_ASSIGNED_CONTEXT ( ( #4207 ) ) GLOBAL_UNIT_ASSIGNED_CONTEXT ( ( #2145, #7291, #5513 ) ) REPRESENTATION_CONTEXT ( 'NONE', 'WORKASPACE' ) );
#4362=ORIENTED_EDGE ( 'NONE', *, *, #150, .F. ) ;
#4371=EDGE_LOOP ( 'NONE', ( #7139, #6887, #5252, #4855 ) ) ;
#4375=DIRECTION ( 'NONE',  ( -0.000000000000000000, 1.000000000000000000, -0.000000000000000000 ) ) ;
#4379=DIRECTION ( 'NONE',  ( 0.000000000000000000, 1.000000000000000000, 0.000000000000000000 ) ) ;
#4382=VECTOR ( 'NONE', #6704, 1000.000000000000000 ) ;
#4386=FACE_BOUND ( 'NONE', #147, .T. ) ;
#4394=CARTESIAN_POINT ( 'NONE',  ( 136.6666666666666288, -25.00000000000000000, -159.8500000000001080 ) ) ;
#4395=DIRECTION ( 'NONE',  ( -0.000000000000000000, -1.000000000000000000, -0.000000000000000000 ) ) ;
#4406=CARTESIAN_POINT ( 'NONE',  ( 303.3333333333333144, -20.00000000000000000, 159.8500000000001080 ) ) ;
#4408=ORIENTED_EDGE ( 'NONE', *, *, #5176, .F. ) ;
#4413=DIRECTION ( 'NONE',  ( 1.000000000000000000, 0.000000000000000000, 0.000000000000000000 ) ) ;
#4415=CARTESIAN_POINT ( 'NONE',  ( 136.6666666666666288, -20.00000000000000000, 159.8500000000001080 ) ) ;
#4431=ADVANCED_FACE ( 'NONE', ( #2816 ), #1147, .F. ) ;
#4442=ORIENTED_EDGE ( 'NONE', *, *, #2046, .F. ) ;
#4443=EDGE_LOOP ( 'NONE', ( #2712, #3957, #366, #3603 ) ) ;
#4445=EDGE_LOOP ( 'NONE', ( #6634, #4535 ) ) ;
#4450=EDGE_LOOP ( 'NONE', ( #641, #4259 ) ) ;
#4454=AXIS2_PLACEMENT_3D ( 'NONE', #3928, #1711, #5728 ) ;
#4467=CARTESIAN_POINT ( 'NONE',  ( 303.3333333333333144, -20.00000000000000000, -159.8500000000001080 ) ) ;
#4477=CIRCLE ( 'NONE', #2189, 2.649999999999985700 ) ;
#4485=VERTEX_POINT ( 'NONE', #6570 ) ;
#4490=DIRECTION ( 'NONE',  ( 0.000000000000000000, 0.000000000000000000, -1.000000000000000000 ) ) ;
#4492=VERTEX_POINT ( 'NONE', #5004 ) ;
#4493=DIRECTION ( 'NONE',  ( 0.000000000000000000, 0.000000000000000000, -1.000000000000000000 ) ) ;
#4518=DIRECTION ( 'NONE',  ( -0.000000000000000000, 1.000000000000000000, -0.000000000000000000 ) ) ;
#4522=STYLED_ITEM('',(#7418),#5676);
#4531=CARTESIAN_POINT ( 'NONE',  ( 53.33333333333330017, -20.00000000000000000, -162.5000000000000853 ) ) ;
#4535=ORIENTED_EDGE ( 'NONE', *, *, #3890, .F. ) ;
#4548=DIRECTION ( 'NONE',  ( 0.000000000000000000, 0.000000000000000000, -1.000000000000000000 ) ) ;
#4554=ORIENTED_EDGE ( 'NONE', *, *, #6825, .T. ) ;
#4565=EDGE_CURVE ( 'NONE', #2874, #5656, #2580, .T. ) ;
#4579=FACE_OUTER_BOUND ( 'NONE', #4735, .T. ) ;
#4603=DIRECTION ( 'NONE',  ( -0.000000000000000000, 1.000000000000000000, -0.000000000000000000 ) ) ;
#4614=LINE ( 'NONE', #6312, #277 ) ;
#4628=ORIENTED_EDGE ( 'NONE', *, *, #6098, .F. ) ;
#4640=ORIENTED_EDGE ( 'NONE', *, *, #5444, .F. ) ;
#4642=ORIENTED_EDGE ( 'NONE', *, *, #976, .F. ) ;
#4668=ADVANCED_FACE ( 'NONE', ( #62 ), #346, .F. ) ;
#4674=ADVANCED_FACE ( 'NONE', ( #5077 ), #5039, .F. ) ;
#4676=CARTESIAN_POINT ( 'NONE',  ( 219.9999999999999716, -25.00000000000000000, 165.1500000000000625 ) ) ;
#4688=AXIS2_PLACEMENT_3D ( 'NONE', #2521, #786, #5842 ) ;
#4690=CARTESIAN_POINT ( 'NONE',  ( 136.6666666666666288, -25.00000000000000000, 165.1500000000000625 ) ) ;
#4705=LINE ( 'NONE', #391, #3992 ) ;
#4706=CARTESIAN_POINT ( 'NONE',  ( 219.9999999999999716, -20.00000000000000000, 159.8500000000001080 ) ) ;
#4707=CIRCLE ( 'NONE', #2891, 2.649999999999985700 ) ;
#4715=DIRECTION ( 'NONE',  ( -0.000000000000000000, 1.000000000000000000, -0.000000000000000000 ) ) ;
#4716=DIRECTION ( 'NONE',  ( 0.000000000000000000, 0.000000000000000000, -1.000000000000000000 ) ) ;
#4718=DIRECTION ( 'NONE',  ( 0.000000000000000000, 0.000000000000000000, -1.000000000000000000 ) ) ;
#4728=VECTOR ( 'NONE', #3335, 1000.000000000000000 ) ;
#4733=CIRCLE ( 'NONE', #5446, 2.649999999999985700 ) ;
#4735=EDGE_LOOP ( 'NONE', ( #1803, #219, #3776, #3728 ) ) ;
#4742=FACE_OUTER_BOUND ( 'NONE', #6059, .T. ) ;
#4763=DIRECTION ( 'NONE',  ( 0.000000000000000000, 1.000000000000000000, 0.000000000000000000 ) ) ;
#4771=SHAPE_REPRESENTATION ( 'base plate', ( #1963 ), #6040 ) ;
#4773=ORIENTED_EDGE ( 'NONE', *, *, #6205, .F. ) ;
#4776=CYLINDRICAL_SURFACE ( 'NONE', #517, 2.649999999999985700 ) ;
#4785=LINE ( 'NONE', #7010, #2681 ) ;
#4796=CARTESIAN_POINT ( 'NONE',  ( 470.0000000000000000, -20.00000000000000000, 200.0000000000000000 ) ) ;
#4799=AXIS2_PLACEMENT_3D ( 'NONE', #5532, #6074, #6110 ) ;
#4826=ORIENTED_EDGE ( 'NONE', *, *, #3890, .T. ) ;
#4830=AXIS2_PLACEMENT_3D ( 'NONE', #2415, #1860, #4718 ) ;
#4832=CYLINDRICAL_SURFACE ( 'NONE', #64, 2.649999999999985700 ) ;
#4841=VERTEX_POINT ( 'NONE', #1895 ) ;
#4842=CARTESIAN_POINT ( 'NONE',  ( 53.33333333333330017, -20.00000000000000000, 162.5000000000000853 ) ) ;
#4844=AXIS2_PLACEMENT_3D ( 'NONE', #2251, #3251, #4548 ) ;
#4848=ORIENTED_EDGE ( 'NONE', *, *, #1864, .T. ) ;
#4849=CARTESIAN_POINT ( 'NONE',  ( 303.3333333333333144, -20.00000000000000000, 165.1500000000000625 ) ) ;
#4851=CIRCLE ( 'NONE', #796, 2.649999999999985700 ) ;
#4855=ORIENTED_EDGE ( 'NONE', *, *, #430, .F. ) ;
#4856=CARTESIAN_POINT ( 'NONE',  ( 386.6666666666666288, -20.00000000000000000, -165.1500000000000625 ) ) ;
#4858=DIRECTION ( 'NONE',  ( 0.000000000000000000, 0.000000000000000000, -1.000000000000000000 ) ) ;
#4865=ORIENTED_EDGE ( 'NONE', *, *, #1026, .F. ) ;
#4870=CYLINDRICAL_SURFACE ( 'NONE', #546, 2.649999999999985700 ) ;
#4874=ORIENTED_EDGE ( 'NONE', *, *, #3511, .F. ) ;
#4880=EDGE_CURVE ( 'NONE', #3696, #6618, #4195, .T. ) ;
#4887=FACE_OUTER_BOUND ( 'NONE', #6947, .T. ) ;
#4899=ORIENTED_EDGE ( 'NONE', *, *, #6992, .F. ) ;
#4900=FACE_BOUND ( 'NONE', #5385, .T. ) ;
#4920=DIRECTION ( 'NONE',  ( 1.000000000000000000, 0.000000000000000000, 0.000000000000000000 ) ) ;
#4923=ADVANCED_FACE ( 'NONE', ( #1424 ), #1977, .T. ) ;
#4944=CIRCLE ( 'NONE', #6984, 2.649999999999985700 ) ;
#4960=ORIENTED_EDGE ( 'NONE', *, *, #5609, .T. ) ;
#4961=VECTOR ( 'NONE', #2847, 1000.000000000000000 ) ;
#4964=CARTESIAN_POINT ( 'NONE',  ( 470.0000000000000000, -25.00000000000000000, 200.0000000000000000 ) ) ;
#4983=FACE_BOUND ( 'NONE', #488, .T. ) ;
#4993=VERTEX_POINT ( 'NONE', #6044 ) ;
#4996=CARTESIAN_POINT ( 'NONE',  ( 136.6666666666666288, -25.00000000000000000, -162.5000000000000853 ) ) ;
#5004=CARTESIAN_POINT ( 'NONE',  ( 470.0000000000000000, -25.00000000000000000, 200.0000000000000000 ) ) ;
#5013=EDGE_LOOP ( 'NONE', ( #1340, #5137 ) ) ;
#5022=LINE ( 'NONE', #5101, #1258 ) ;
#5039=CYLINDRICAL_SURFACE ( 'NONE', #3967, 2.649999999999985700 ) ;
#5040=FACE_OUTER_BOUND ( 'NONE', #6913, .T. ) ;
#5047=ORIENTED_EDGE ( 'NONE', *, *, #3283, .F. ) ;
#5067=CARTESIAN_POINT ( 'NONE',  ( 386.6666666666666288, -20.00000000000000000, 162.5000000000000853 ) ) ;
#5077=FACE_OUTER_BOUND ( 'NONE', #5569, .T. ) ;
#5090=ORIENTED_EDGE ( 'NONE', *, *, #1730, .F. ) ;
#5100=FACE_BOUND ( 'NONE', #2538, .T. ) ;
#5101=CARTESIAN_POINT ( 'NONE',  ( 470.0000000000000000, -20.00000000000000000, 200.0000000000000000 ) ) ;
#5108=DIRECTION ( 'NONE',  ( -0.000000000000000000, 1.000000000000000000, -0.000000000000000000 ) ) ;
#5117=DIRECTION ( 'NONE',  ( 0.000000000000000000, 0.000000000000000000, 1.000000000000000000 ) ) ;
#5128=VERTEX_POINT ( 'NONE', #6263 ) ;
#5131=FACE_BOUND ( 'NONE', #1515, .T. ) ;
#5137=ORIENTED_EDGE ( 'NONE', *, *, #430, .T. ) ;
#5145=CARTESIAN_POINT ( 'NONE',  ( 303.3333333333333144, -20.00000000000000000, 162.5000000000000853 ) ) ;
#5162=EDGE_CURVE ( 'NONE', #6179, #4054, #1900, .T. ) ;
#5166=CIRCLE ( 'NONE', #4688, 2.649999999999985700 ) ;
#5176=EDGE_CURVE ( 'NONE', #4054, #6179, #4301, .T. ) ;
#5181=LINE ( 'NONE', #3552, #6635 ) ;
#5185=PRODUCT_DEFINITION_FORMATION_WITH_SPECIFIED_SOURCE ( 'ANY', '', #3544, .NOT_KNOWN. ) ;
#5187=CIRCLE ( 'NONE', #758, 2.649999999999985700 ) ;
#5189=ORIENTED_EDGE ( 'NONE', *, *, #1510, .T. ) ;
#5195=COLOUR_RGB ( '',0.8941176470588234615, 0.8941176470588234615, 0.8941176470588234615 ) ;
#5229=CARTESIAN_POINT ( 'NONE',  ( 0.000000000000000000, 0.000000000000000000, 200.0000000000000000 ) ) ;
#5230=ORIENTED_EDGE ( 'NONE', *, *, #5176, .T. ) ;
#5252=ORIENTED_EDGE ( 'NONE', *, *, #2473, .T. ) ;
#5253=VERTEX_POINT ( 'NONE', #6369 ) ;
#5269=EDGE_CURVE ( 'NONE', #3098, #847, #1269, .T. ) ;
#5280=ORIENTED_EDGE ( 'NONE', *, *, #5940, .F. ) ;
#5286=CIRCLE ( 'NONE', #6386, 2.649999999999985700 ) ;
#5290=AXIS2_PLACEMENT_3D ( 'NONE', #5441, #2113, #6015 ) ;
#5304=AXIS2_PLACEMENT_3D ( 'NONE', #6005, #3633, #4276 ) ;
#5308=ORIENTED_EDGE ( 'NONE', *, *, #6583, .T. ) ;
#5326=CARTESIAN_POINT ( 'NONE',  ( 386.6666666666666288, -25.00000000000000000, 162.5000000000000853 ) ) ;
#5329=ORIENTED_EDGE ( 'NONE', *, *, #6128, .T. ) ;
#5337=AXIS2_PLACEMENT_3D ( 'NONE', #3599, #5903, #3031 ) ;
#5344=EDGE_CURVE ( 'NONE', #7189, #2910, #5286, .T. ) ;
#5351=ADVANCED_FACE ( 'NONE', ( #1379 ), #3771, .F. ) ;
#5362=EDGE_LOOP ( 'NONE', ( #5426, #4001, #835, #179 ) ) ;
#5370=DIRECTION ( 'NONE',  ( 0.000000000000000000, 0.000000000000000000, 1.000000000000000000 ) ) ;
#5374=ORIENTED_EDGE ( 'NONE', *, *, #5680, .T. ) ;
#5382=AXIS2_PLACEMENT_3D ( 'NONE', #996, #3210, #5512 ) ;
#5383=FACE_BOUND ( 'NONE', #3621, .T. ) ;
#5385=EDGE_LOOP ( 'NONE', ( #2372, #2337 ) ) ;
#5386=VERTEX_POINT ( 'NONE', #4856 ) ;
#5401=EDGE_CURVE ( 'NONE', #1772, #6816, #6109, .T. ) ;
#5407=DIRECTION ( 'NONE',  ( 0.000000000000000000, 0.000000000000000000, 1.000000000000000000 ) ) ;
#5411=ORIENTED_EDGE ( 'NONE', *, *, #2268, .F. ) ;
#5419=ORIENTED_EDGE ( 'NONE', *, *, #7274, .T. ) ;
#5423=CIRCLE ( 'NONE', #420, 2.649999999999985700 ) ;
#5425=ORIENTED_EDGE ( 'NONE', *, *, #4880, .T. ) ;
#5426=ORIENTED_EDGE ( 'NONE', *, *, #1466, .F. ) ;
#5427=DIRECTION ( 'NONE',  ( 1.000000000000000000, 0.000000000000000000, -0.000000000000000000 ) ) ;
#5439=VECTOR ( 'NONE', #7336, 1000.000000000000000 ) ;
#5441=CARTESIAN_POINT ( 'NONE',  ( 386.6666666666666288, -20.00000000000000000, 162.5000000000000853 ) ) ;
#5444=EDGE_CURVE ( 'NONE', #3280, #6176, #302, .T. ) ;
#5446=AXIS2_PLACEMENT_3D ( 'NONE', #4996, #7311, #3240 ) ;
#5447=ORIENTED_EDGE ( 'NONE', *, *, #5401, .F. ) ;
#5464=LINE ( 'NONE', #1508, #1587 ) ;
#5468=LINE ( 'NONE', #2614, #7241 ) ;
#5507=CARTESIAN_POINT ( 'NONE',  ( 136.6666666666666288, -25.00000000000000000, -162.5000000000000853 ) ) ;
#5512=DIRECTION ( 'NONE',  ( 0.000000000000000000, 0.000000000000000000, 1.000000000000000000 ) ) ;
#5513=( NAMED_UNIT ( * ) SI_UNIT ( $, .STERADIAN. ) SOLID_ANGLE_UNIT ( ) );
#5532=CARTESIAN_POINT ( 'NONE',  ( 53.33333333333330017, -20.00000000000000000, -162.5000000000000853 ) ) ;
#5542=VECTOR ( 'NONE', #3102, 1000.000000000000000 ) ;
#5552=AXIS2_PLACEMENT_3D ( 'NONE', #7319, #2318, #585 ) ;
#5553=AXIS2_PLACEMENT_3D ( 'NONE', #7264, #3720, #3844 ) ;
#5555=CARTESIAN_POINT ( 'NONE',  ( 386.6666666666666288, -20.00000000000000000, 159.8500000000001080 ) ) ;
#5556=VERTEX_POINT ( 'NONE', #2196 ) ;
#5569=EDGE_LOOP ( 'NONE', ( #1504, #3610, #5594, #4362 ) ) ;
#5572=ADVANCED_FACE ( 'NONE', ( #5577, #6301, #4983, #6254, #1015, #1121, #5100, #3394, #6188, #5131, #3274 ), #2159, .T. ) ;
#5576=ORIENTED_EDGE ( 'NONE', *, *, #5758, .F. ) ;
#5577=FACE_BOUND ( 'NONE', #348, .T. ) ;
#5586=DIRECTION ( 'NONE',  ( 0.000000000000000000, 0.000000000000000000, 1.000000000000000000 ) ) ;
#5594=ORIENTED_EDGE ( 'NONE', *, *, #521, .T. ) ;
#5596=EDGE_CURVE ( 'NONE', #1179, #4485, #2123, .T. ) ;
#5600=SHAPE_REPRESENTATION_RELATIONSHIP ( 'NONE' , 'NONE' ,  #4771, #2710 ) ;
#5609=EDGE_CURVE ( 'NONE', #3098, #647, #3481, .T. ) ;
#5627=CYLINDRICAL_SURFACE ( 'NONE', #421, 2.649999999999985700 ) ;
#5631=CYLINDRICAL_SURFACE ( 'NONE', #4844, 2.649999999999985700 ) ;
#5655=ORIENTED_EDGE ( 'NONE', *, *, #5982, .T. ) ;
#5656=VERTEX_POINT ( 'NONE', #7132 ) ;
#5665=DIRECTION ( 'NONE',  ( -0.000000000000000000, 1.000000000000000000, -0.000000000000000000 ) ) ;
#5673=CIRCLE ( 'NONE', #4218, 2.649999999999985700 ) ;
#5676=MANIFOLD_SOLID_BREP ( 'Mirror1', #6149 ) ;
#5680=EDGE_CURVE ( 'NONE', #1772, #432, #1643, .T. ) ;
#5682=ORIENTED_EDGE ( 'NONE', *, *, #6205, .T. ) ;
#5688=CYLINDRICAL_SURFACE ( 'NONE', #3122, 2.649999999999985700 ) ;
#5690=EDGE_CURVE ( 'NONE', #7294, #847, #3534, .T. ) ;
#5707=FACE_OUTER_BOUND ( 'NONE', #6116, .T. ) ;
#5721=ORIENTED_EDGE ( 'NONE', *, *, #3744, .T. ) ;
#5728=DIRECTION ( 'NONE',  ( 0.000000000000000000, 0.000000000000000000, 1.000000000000000000 ) ) ;
#5737=CARTESIAN_POINT ( 'NONE',  ( 136.6666666666666288, -20.00000000000000000, -159.8500000000001080 ) ) ;
#5741=CYLINDRICAL_SURFACE ( 'NONE', #3623, 2.649999999999985700 ) ;
#5757=PLANE ( 'NONE',  #5337 ) ;
#5758=EDGE_CURVE ( 'NONE', #6697, #4492, #6655, .T. ) ;
#5767=CARTESIAN_POINT ( 'NONE',  ( 53.33333333333330017, -20.00000000000000000, 165.1500000000000625 ) ) ;
#5791=ORIENTED_EDGE ( 'NONE', *, *, #5596, .T. ) ;
#5793=APPLICATION_CONTEXT ( 'automotive_design' ) ;
#5800=DIRECTION ( 'NONE',  ( 0.000000000000000000, 0.000000000000000000, 1.000000000000000000 ) ) ;
#5801=ORIENTED_EDGE ( 'NONE', *, *, #680, .T. ) ;
#5805=CARTESIAN_POINT ( 'NONE',  ( 136.6666666666666288, -20.00000000000000000, 162.5000000000000853 ) ) ;
#5813=EDGE_CURVE ( 'NONE', #1784, #1652, #4069, .T. ) ;
#5818=DIRECTION ( 'NONE',  ( 1.000000000000000000, 0.000000000000000000, 0.000000000000000000 ) ) ;
#5824=ORIENTED_EDGE ( 'NONE', *, *, #150, .T. ) ;
#5829=DIRECTION ( 'NONE',  ( 1.000000000000000000, 0.000000000000000000, 0.000000000000000000 ) ) ;
#5830=MECHANICAL_DESIGN_GEOMETRIC_PRESENTATION_REPRESENTATION('',(#4522),#334);
#5833=EDGE_LOOP ( 'NONE', ( #1047, #1062, #653, #4773 ) ) ;
#5834=EDGE_CURVE ( 'NONE', #3333, #2910, #6880, .T. ) ;
#5836=LINE ( 'NONE', #4706, #3145 ) ;
#5842=DIRECTION ( 'NONE',  ( 0.000000000000000000, 0.000000000000000000, -1.000000000000000000 ) ) ;
#5846=DIRECTION ( 'NONE',  ( -0.000000000000000000, 1.000000000000000000, -0.000000000000000000 ) ) ;
#5893=ORIENTED_EDGE ( 'NONE', *, *, #2057, .F. ) ;
#5901=CIRCLE ( 'NONE', #2998, 2.649999999999985700 ) ;
#5903=DIRECTION ( 'NONE',  ( 0.000000000000000000, 0.000000000000000000, -1.000000000000000000 ) ) ;
#5905=VECTOR ( 'NONE', #911, 1000.000000000000000 ) ;
#5906=EDGE_CURVE ( 'NONE', #2399, #153, #5181, .T. ) ;
#5907=ORIENTED_EDGE ( 'NONE', *, *, #4565, .T. ) ;
#5924=EDGE_LOOP ( 'NONE', ( #6389, #1540 ) ) ;
#5930=DIRECTION ( 'NONE',  ( 0.000000000000000000, 0.000000000000000000, -1.000000000000000000 ) ) ;
#5936=VECTOR ( 'NONE', #1134, 1000.000000000000000 ) ;
#5940=EDGE_CURVE ( 'NONE', #5999, #3484, #1148, .T. ) ;
#5954=CARTESIAN_POINT ( 'NONE',  ( 303.3333333333333144, -20.00000000000000000, -165.1500000000000625 ) ) ;
#5956=FACE_OUTER_BOUND ( 'NONE', #2342, .T. ) ;
#5959=EDGE_LOOP ( 'NONE', ( #4874, #2139 ) ) ;
#5960=DIRECTION ( 'NONE',  ( 0.000000000000000000, 0.000000000000000000, 1.000000000000000000 ) ) ;
#5982=EDGE_CURVE ( 'NONE', #450, #541, #2075, .T. ) ;
#5999=VERTEX_POINT ( 'NONE', #802 ) ;
#6001=CARTESIAN_POINT ( 'NONE',  ( 303.3333333333333144, -25.00000000000000000, -165.1500000000000625 ) ) ;
#6005=CARTESIAN_POINT ( 'NONE',  ( 303.3333333333333144, -25.00000000000000000, 162.5000000000000853 ) ) ;
#6014=SURFACE_SIDE_STYLE ('',( #4284 ) ) ;
#6015=DIRECTION ( 'NONE',  ( 0.000000000000000000, 0.000000000000000000, 1.000000000000000000 ) ) ;
#6029=AXIS2_PLACEMENT_3D ( 'NONE', #6517, #4379, #2037 ) ;
#6035=CARTESIAN_POINT ( 'NONE',  ( 136.6666666666666288, -20.00000000000000000, -165.1500000000000625 ) ) ;
#6040=( GEOMETRIC_REPRESENTATION_CONTEXT ( 3 ) GLOBAL_UNCERTAINTY_ASSIGNED_CONTEXT ( ( #1366 ) ) GLOBAL_UNIT_ASSIGNED_CONTEXT ( ( #2021, #3065, #287 ) ) REPRESENTATION_CONTEXT ( 'NONE', 'WORKASPACE' ) );
#6043=ORIENTED_EDGE ( 'NONE', *, *, #849, .F. ) ;
#6044=CARTESIAN_POINT ( 'NONE',  ( 219.9999999999999716, -20.00000000000000000, -165.1500000000000625 ) ) ;
#6059=EDGE_LOOP ( 'NONE', ( #1456, #1177, #6236, #1999 ) ) ;
#6074=DIRECTION ( 'NONE',  ( 0.000000000000000000, 1.000000000000000000, 0.000000000000000000 ) ) ;
#6089=ADVANCED_FACE ( 'NONE', ( #1247 ), #4832, .F. ) ;
#6098=EDGE_CURVE ( 'NONE', #2399, #2352, #1137, .T. ) ;
#6109=LINE ( 'NONE', #5954, #3121 ) ;
#6110=DIRECTION ( 'NONE',  ( 0.000000000000000000, 0.000000000000000000, -1.000000000000000000 ) ) ;
#6111=FACE_OUTER_BOUND ( 'NONE', #333, .T. ) ;
#6113=ORIENTED_EDGE ( 'NONE', *, *, #1453, .F. ) ;
#6115=AXIS2_PLACEMENT_3D ( 'NONE', #5067, #579, #5586 ) ;
#6116=EDGE_LOOP ( 'NONE', ( #2442, #40, #1961, #7128 ) ) ;
#6121=CARTESIAN_POINT ( 'NONE',  ( 470.0000000000000000, -20.00000000000000000, -200.0000000000000000 ) ) ;
#6124=LINE ( 'NONE', #5555, #5905 ) ;
#6128=EDGE_CURVE ( 'NONE', #3198, #5656, #3165, .T. ) ;
#6149=CLOSED_SHELL ( 'NONE', ( #7330, #4431, #5351, #1600, #2612, #4668, #3793, #4674, #6089, #2242, #2949, #4923, #5572, #7231, #1206, #1275, #3052, #2650, #6646, #2483, #6693, #3962, #4065, #143, #4142, #6187 ) ) ;
#6161=DIRECTION ( 'NONE',  ( 0.000000000000000000, 0.000000000000000000, -1.000000000000000000 ) ) ;
#6176=VERTEX_POINT ( 'NONE', #6121 ) ;
#6179=VERTEX_POINT ( 'NONE', #317 ) ;
#6185=ORIENTED_EDGE ( 'NONE', *, *, #1164, .F. ) ;
#6187=ADVANCED_FACE ( 'NONE', ( #2012 ), #4870, .F. ) ;
#6188=FACE_BOUND ( 'NONE', #5924, .T. ) ;
#6189=DIRECTION ( 'NONE',  ( 0.000000000000000000, 1.000000000000000000, 0.000000000000000000 ) ) ;
#6205=EDGE_CURVE ( 'NONE', #153, #4993, #3628, .T. ) ;
#6208=CARTESIAN_POINT ( 'NONE',  ( 53.33333333333330017, -25.00000000000000000, 162.5000000000000853 ) ) ;
#6212=EDGE_LOOP ( 'NONE', ( #1261, #570, #791, #2224 ) ) ;
#6236=ORIENTED_EDGE ( 'NONE', *, *, #7004, .F. ) ;
#6238=DIRECTION ( 'NONE',  ( 0.000000000000000000, 1.000000000000000000, 0.000000000000000000 ) ) ;
#6243=AXIS2_PLACEMENT_3D ( 'NONE', #1663, #1695, #3334 ) ;
#6248=CARTESIAN_POINT ( 'NONE',  ( 470.0000000000000000, -20.00000000000000000, -200.0000000000000000 ) ) ;
#6254=FACE_BOUND ( 'NONE', #5013, .T. ) ;
#6263=CARTESIAN_POINT ( 'NONE',  ( 136.6666666666666288, -25.00000000000000000, -165.1500000000000625 ) ) ;
#6264=CARTESIAN_POINT ( 'NONE',  ( 136.6666666666666288, -20.00000000000000000, -165.1500000000000625 ) ) ;
#6287=ORIENTED_EDGE ( 'NONE', *, *, #2824, .T. ) ;
#6288=ORIENTED_EDGE ( 'NONE', *, *, #1730, .T. ) ;
#6296=DIRECTION ( 'NONE',  ( 0.000000000000000000, 0.000000000000000000, -1.000000000000000000 ) ) ;
#6297=AXIS2_PLACEMENT_3D ( 'NONE', #1914, #3804, #5407 ) ;
#6301=FACE_BOUND ( 'NONE', #2841, .T. ) ;
#6305=ORIENTED_EDGE ( 'NONE', *, *, #680, .F. ) ;
#6312=CARTESIAN_POINT ( 'NONE',  ( 386.6666666666666288, -20.00000000000000000, -159.8500000000001080 ) ) ;
#6343=CARTESIAN_POINT ( 'NONE',  ( 53.33333333333330017, -20.00000000000000000, -162.5000000000000853 ) ) ;
#6346=CARTESIAN_POINT ( 'NONE',  ( 219.9999999999999716, -20.00000000000000000, 159.8500000000001080 ) ) ;
#6369=CARTESIAN_POINT ( 'NONE',  ( 386.6666666666666288, -20.00000000000000000, -159.8500000000001080 ) ) ;
#6375=ORIENTED_EDGE ( 'NONE', *, *, #5269, .T. ) ;
#6380=CARTESIAN_POINT ( 'NONE',  ( -30.00000000000002842, -20.00000000000000000, -200.0000000000000000 ) ) ;
#6386=AXIS2_PLACEMENT_3D ( 'NONE', #5805, #4715, #119 ) ;
#6389=ORIENTED_EDGE ( 'NONE', *, *, #2824, .F. ) ;
#6395=AXIS2_PLACEMENT_3D ( 'NONE', #2465, #1898, #4194 ) ;
#6417=UNCERTAINTY_MEASURE_WITH_UNIT (LENGTH_MEASURE( 1.000000000000000082E-05 ), #4283, 'distance_accuracy_value', 'NONE');
#6418=ORIENTED_EDGE ( 'NONE', *, *, #3562, .T. ) ;
#6419=AXIS2_PLACEMENT_3D ( 'NONE', #2010, #2531, #5930 ) ;
#6433=DIRECTION ( 'NONE',  ( -1.000000000000000000, 0.000000000000000000, -0.000000000000000000 ) ) ;
#6434=EDGE_LOOP ( 'NONE', ( #5655, #1578 ) ) ;
#6436=CARTESIAN_POINT ( 'NONE',  ( 53.33333333333330017, -25.00000000000000000, 159.8500000000001080 ) ) ;
#6505=ORIENTED_EDGE ( 'NONE', *, *, #462, .F. ) ;
#6508=AXIS2_PLACEMENT_3D ( 'NONE', #5326, #4763, #1349 ) ;
#6517=CARTESIAN_POINT ( 'NONE',  ( 303.3333333333333144, -20.00000000000000000, -162.5000000000000853 ) ) ;
#6562=ORIENTED_EDGE ( 'NONE', *, *, #7297, .T. ) ;
#6570=CARTESIAN_POINT ( 'NONE',  ( 53.33333333333330017, -20.00000000000000000, -165.1500000000000625 ) ) ;
#6575=ORIENTED_EDGE ( 'NONE', *, *, #3562, .F. ) ;
#6581=EDGE_CURVE ( 'NONE', #4993, #153, #891, .T. ) ;
#6583=EDGE_CURVE ( 'NONE', #6697, #2874, #4785, .T. ) ;
#6584=DIRECTION ( 'NONE',  ( -0.000000000000000000, -0.000000000000000000, -1.000000000000000000 ) ) ;
#6586=DIRECTION ( 'NONE',  ( -0.000000000000000000, 1.000000000000000000, -0.000000000000000000 ) ) ;
#6597=DIRECTION ( 'NONE',  ( 0.000000000000000000, 0.000000000000000000, 1.000000000000000000 ) ) ;
#6607=ORIENTED_EDGE ( 'NONE', *, *, #2473, .F. ) ;
#6618=VERTEX_POINT ( 'NONE', #6035 ) ;
#6628=VECTOR ( 'NONE', #3204, 1000.000000000000000 ) ;
#6634=ORIENTED_EDGE ( 'NONE', *, *, #5680, .F. ) ;
#6635=VECTOR ( 'NONE', #659, 1000.000000000000000 ) ;
#6646=ADVANCED_FACE ( 'NONE', ( #7113 ), #1970, .F. ) ;
#6648=CYLINDRICAL_SURFACE ( 'NONE', #1603, 2.649999999999985700 ) ;
#6655=LINE ( 'NONE', #2620, #6720 ) ;
#6674=DIRECTION ( 'NONE',  ( 0.000000000000000000, 0.000000000000000000, 1.000000000000000000 ) ) ;
#6677=DIRECTION ( 'NONE',  ( 0.000000000000000000, -0.000000000000000000, 1.000000000000000000 ) ) ;
#6680=ORIENTED_EDGE ( 'NONE', *, *, #5834, .T. ) ;
#6693=ADVANCED_FACE ( 'NONE', ( #6111 ), #3851, .F. ) ;
#6697=VERTEX_POINT ( 'NONE', #3193 ) ;
#6703=LINE ( 'NONE', #3267, #5542 ) ;
#6704=DIRECTION ( 'NONE',  ( -0.000000000000000000, 1.000000000000000000, -0.000000000000000000 ) ) ;
#6712=FACE_BOUND ( 'NONE', #7191, .T. ) ;
#6720=VECTOR ( 'NONE', #4920, 1000.000000000000000 ) ;
#6736=VECTOR ( 'NONE', #6856, 1000.000000000000000 ) ;
#6739=CARTESIAN_POINT ( 'NONE',  ( 53.33333333333330017, -20.00000000000000000, 159.8500000000001080 ) ) ;
#6740=AXIS2_PLACEMENT_3D ( 'NONE', #7050, #723, #2977 ) ;
#6762=CARTESIAN_POINT ( 'NONE',  ( 386.6666666666666288, -20.00000000000000000, -162.5000000000000853 ) ) ;
#6782=CARTESIAN_POINT ( 'NONE',  ( 303.3333333333333144, -20.00000000000000000, -162.5000000000000853 ) ) ;
#6785=DIRECTION ( 'NONE',  ( -0.000000000000000000, 1.000000000000000000, -0.000000000000000000 ) ) ;
#6816=VERTEX_POINT ( 'NONE', #3353 ) ;
#6825=EDGE_CURVE ( 'NONE', #3661, #3696, #1124, .T. ) ;
#6852=VECTOR ( 'NONE', #1174, 1000.000000000000000 ) ;
#6856=DIRECTION ( 'NONE',  ( 0.000000000000000000, 1.000000000000000000, 0.000000000000000000 ) ) ;
#6864=CARTESIAN_POINT ( 'NONE',  ( 386.6666666666666288, -20.00000000000000000, 162.5000000000000853 ) ) ;
#6872=AXIS2_PLACEMENT_3D ( 'NONE', #7162, #2615, #3128 ) ;
#6880=LINE ( 'NONE', #1767, #7229 ) ;
#6887=ORIENTED_EDGE ( 'NONE', *, *, #849, .T. ) ;
#6890=EDGE_CURVE ( 'NONE', #3280, #4492, #5022, .T. ) ;
#6892=DIRECTION ( 'NONE',  ( 0.000000000000000000, 1.000000000000000000, 0.000000000000000000 ) ) ;
#6904=CIRCLE ( 'NONE', #3780, 2.649999999999985700 ) ;
#6913=EDGE_LOOP ( 'NONE', ( #5801, #4227, #6185, #6607 ) ) ;
#6924=EDGE_LOOP ( 'NONE', ( #4960, #1709 ) ) ;
#6947=EDGE_LOOP ( 'NONE', ( #3134, #2812, #5308, #5907 ) ) ;
#6968=ORIENTED_EDGE ( 'NONE', *, *, #1510, .F. ) ;
#6984=AXIS2_PLACEMENT_3D ( 'NONE', #2499, #243, #912 ) ;
#6987=CARTESIAN_POINT ( 'NONE',  ( 303.3333333333333144, -25.00000000000000000, 162.5000000000000853 ) ) ;
#6992=EDGE_CURVE ( 'NONE', #3333, #1043, #7114, .T. ) ;
#6997=DIRECTION ( 'NONE',  ( 0.000000000000000000, 0.000000000000000000, -1.000000000000000000 ) ) ;
#7003=ORIENTED_EDGE ( 'NONE', *, *, #6581, .T. ) ;
#7004=EDGE_CURVE ( 'NONE', #2874, #3280, #2369, .T. ) ;
#7007=DIRECTION ( 'NONE',  ( -0.000000000000000000, -1.000000000000000000, -0.000000000000000000 ) ) ;
#7010=CARTESIAN_POINT ( 'NONE',  ( -30.00000000000002842, -25.00000000000000000, 200.0000000000000000 ) ) ;
#7037=DIRECTION ( 'NONE',  ( -0.000000000000000000, 1.000000000000000000, -0.000000000000000000 ) ) ;
#7050=CARTESIAN_POINT ( 'NONE',  ( 53.33333333333330017, -20.00000000000000000, 162.5000000000000853 ) ) ;
#7053=CARTESIAN_POINT ( 'NONE',  ( 386.6666666666666288, -25.00000000000000000, 162.5000000000000853 ) ) ;
#7060=EDGE_CURVE ( 'NONE', #763, #1652, #5836, .T. ) ;
#7096=ORIENTED_EDGE ( 'NONE', *, *, #5401, .T. ) ;
#7113=FACE_OUTER_BOUND ( 'NONE', #3838, .T. ) ;
#7114=CIRCLE ( 'NONE', #1845, 2.649999999999985700 ) ;
#7116=DIRECTION ( 'NONE',  ( 0.000000000000000000, 1.000000000000000000, 0.000000000000000000 ) ) ;
#7127=CIRCLE ( 'NONE', #6419, 2.649999999999985700 ) ;
#7128=ORIENTED_EDGE ( 'NONE', *, *, #5834, .F. ) ;
#7132=CARTESIAN_POINT ( 'NONE',  ( -30.00000000000002842, -20.00000000000000000, -200.0000000000000000 ) ) ;
#7133=AXIS2_PLACEMENT_3D ( 'NONE', #5229, #2474, #6433 ) ;
#7139=ORIENTED_EDGE ( 'NONE', *, *, #3712, .F. ) ;
#7148=CARTESIAN_POINT ( 'NONE',  ( 386.6666666666666288, -20.00000000000000000, 159.8500000000001080 ) ) ;
#7152=FACE_BOUND ( 'NONE', #3161, .T. ) ;
#7159=DIRECTION ( 'NONE',  ( 0.000000000000000000, 0.000000000000000000, -1.000000000000000000 ) ) ;
#7161=FACE_OUTER_BOUND ( 'NONE', #126, .T. ) ;
#7162=CARTESIAN_POINT ( 'NONE',  ( 219.9999999999999716, -20.00000000000000000, 162.5000000000000853 ) ) ;
#7189=VERTEX_POINT ( 'NONE', #4289 ) ;
#7191=EDGE_LOOP ( 'NONE', ( #3797, #4628 ) ) ;
#7210=ORIENTED_EDGE ( 'NONE', *, *, #7060, .F. ) ;
#7219=CARTESIAN_POINT ( 'NONE',  ( 303.3333333333333144, -20.00000000000000000, 162.5000000000000853 ) ) ;
#7229=VECTOR ( 'NONE', #3479, 1000.000000000000000 ) ;
#7231=ADVANCED_FACE ( 'NONE', ( #4887 ), #2029, .T. ) ;
#7241=VECTOR ( 'NONE', #867, 1000.000000000000000 ) ;
#7243=DIRECTION ( 'NONE',  ( 0.000000000000000000, 0.000000000000000000, 1.000000000000000000 ) ) ;
#7245=VECTOR ( 'NONE', #2929, 1000.000000000000000 ) ;
#7251=CARTESIAN_POINT ( 'NONE',  ( 219.9999999999999716, -25.00000000000000000, 162.5000000000000853 ) ) ;
#7254=VECTOR ( 'NONE', #88, 1000.000000000000000 ) ;
#7260=CIRCLE ( 'NONE', #4256, 2.649999999999985700 ) ;
#7262=DIRECTION ( 'NONE',  ( 0.000000000000000000, 0.000000000000000000, -1.000000000000000000 ) ) ;
#7264=CARTESIAN_POINT ( 'NONE',  ( 303.3333333333333144, -20.00000000000000000, -162.5000000000000853 ) ) ;
#7265=LINE ( 'NONE', #4415, #4382 ) ;
#7269=DIRECTION ( 'NONE',  ( 0.000000000000000000, 0.000000000000000000, 1.000000000000000000 ) ) ;
#7273=ORIENTED_EDGE ( 'NONE', *, *, #416, .F. ) ;
#7274=EDGE_CURVE ( 'NONE', #3198, #3944, #2823, .T. ) ;
#7277=LINE ( 'NONE', #3361, #1746 ) ;
#7279=CARTESIAN_POINT ( 'NONE',  ( -30.00000000000002842, -25.00000000000000000, -200.0000000000000000 ) ) ;
#7281=DIRECTION ( 'NONE',  ( -0.000000000000000000, -1.000000000000000000, -0.000000000000000000 ) ) ;
#7286=DIRECTION ( 'NONE',  ( -0.000000000000000000, -0.000000000000000000, -1.000000000000000000 ) ) ;
#7291=( NAMED_UNIT ( * ) PLANE_ANGLE_UNIT ( ) SI_UNIT ( $, .RADIAN. ) );
#7294=VERTEX_POINT ( 'NONE', #6739 ) ;
#7297=EDGE_CURVE ( 'NONE', #6176, #3944, #2851, .T. ) ;
#7311=DIRECTION ( 'NONE',  ( -0.000000000000000000, -1.000000000000000000, -0.000000000000000000 ) ) ;
#7319=CARTESIAN_POINT ( 'NONE',  ( 53.33333333333330017, -25.00000000000000000, -162.5000000000000853 ) ) ;
#7325=DIRECTION ( 'NONE',  ( 0.000000000000000000, 1.000000000000000000, 0.000000000000000000 ) ) ;
#7330=ADVANCED_FACE ( 'NONE', ( #3346 ), #5688, .F. ) ;
#7332=VERTEX_POINT ( 'NONE', #2153 ) ;
#7336=DIRECTION ( 'NONE',  ( 0.000000000000000000, -1.000000000000000000, 0.000000000000000000 ) ) ;
#7412=COLOUR_RGB('Dark Blue',0.08,0.2,0.34);
#7413=FILL_AREA_STYLE_COLOUR('',#7412);
#7414=FILL_AREA_STYLE('',(#7413));
#7415=SURFACE_STYLE_FILL_AREA(#7414);
#7416=SURFACE_SIDE_STYLE('',(#7415));
#7417=SURFACE_STYLE_USAGE(.BOTH.,#7416);
#7418=PRESENTATION_STYLE_ASSIGNMENT((#7417));
ENDSEC;
END-ISO-10303-21;
